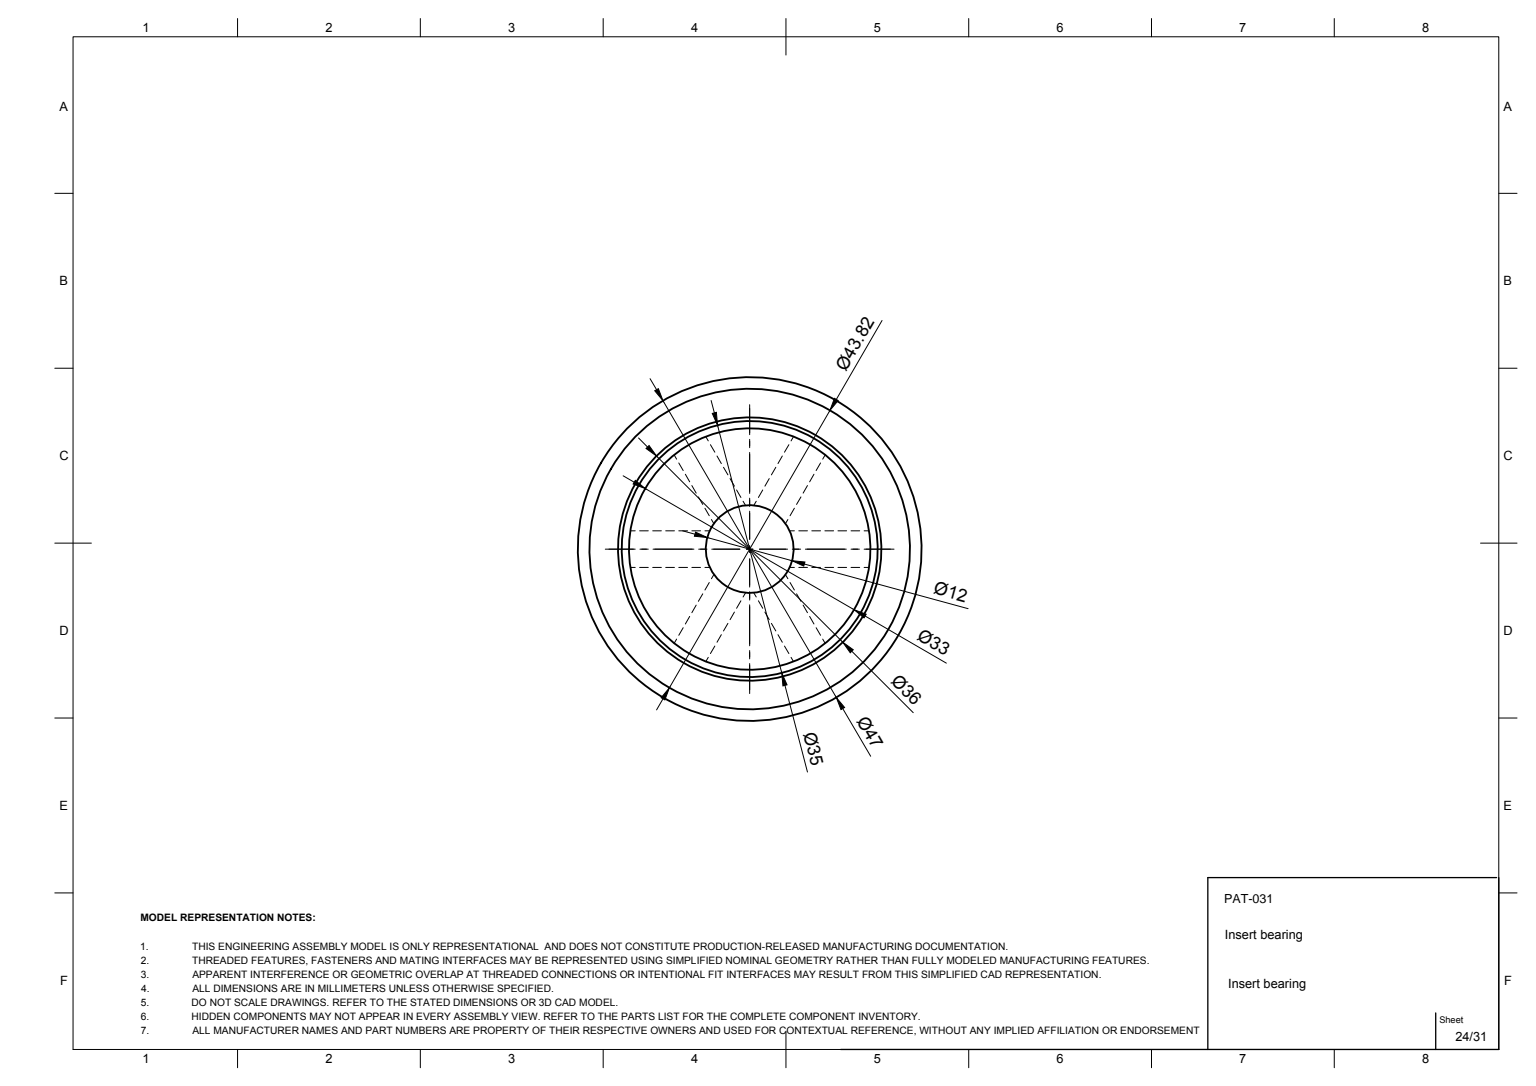
ISO-10303-21;
HEADER;
/* Generated by software containing ST-Developer
 * from STEP Tools, Inc. (www.steptools.com) 
 */

FILE_DESCRIPTION(
/* description */ ('Double-row support with tensioned shaft'),
/* implementation_level */ '2;1');

FILE_NAME(
/* name */ 'Insert bearing.step',
/* time_stamp */ '2026-10-27T10:50:35-07:00',
/* author */ (''),
/* organization */ (''),
/* preprocessor_version */ 'ST-DEVELOPER v20.2',
/* originating_system */ 'Autodesk Translation Framework v15.17.0.0',
/* authorisation */ '');

FILE_SCHEMA (('AUTOMOTIVE_DESIGN { 1 0 10303 214 3 1 1 }'));
ENDSEC;

DATA;
#10=MECHANICAL_DESIGN_GEOMETRIC_PRESENTATION_REPRESENTATION('',(#499,#500),#11559);
#363=B_SPLINE_CURVE_WITH_KNOTS('',3,(#10336,#10337,#10338,#10339,#10340,
#10341,#10342,#10343,#10344,#10345),.UNSPECIFIED.,.F.,.F.,(4,2,2,2,4),(1.13193471301885,
1.22626174930539,1.32058878559194,1.41491753480854,1.50924628402513),
 .UNSPECIFIED.);
#364=B_SPLINE_CURVE_WITH_KNOTS('',3,(#10347,#10348,#10349,#10350,#10351,
#10352,#10353,#10354,#10355,#10356,#10357,#10358,#10359,#10360,#10361,#10362,
#10363,#10364),.UNSPECIFIED.,.F.,.F.,(4,2,2,2,2,2,2,2,4),(0.377311571006283,
0.471638607292829,0.565965643579376,0.66029439279597,0.754623142012565,
0.84895189122916,0.943280640445754,1.0376076767323,1.13193471301885),
 .UNSPECIFIED.);
#365=B_SPLINE_CURVE_WITH_KNOTS('',3,(#10365,#10366,#10367,#10368,#10369,
#10370,#10371,#10372,#10373,#10374),.UNSPECIFIED.,.F.,.F.,(4,2,2,2,4),(1.50924628402513,
1.60357503324173,1.69790378245832,1.79223081874487,1.88655785503141),
 .UNSPECIFIED.);
#366=B_SPLINE_CURVE_WITH_KNOTS('',3,(#10377,#10378,#10379,#10380,#10381,
#10382,#10383,#10384,#10385,#10386,#10387,#10388,#10389,#10390,#10391,#10392,
#10393,#10394,#10395,#10396,#10397,#10398,#10399,#10400,#10401,#10402,#10403,
#10404,#10405,#10406,#10407,#10408,#10409,#10410),.UNSPECIFIED.,.T.,.F.,
(4,2,2,2,2,2,2,2,2,2,2,2,2,2,2,2,4),(0.,0.0955080856649705,0.191016171329941,
0.286408845249646,0.38180151916935,0.477194193089055,0.572586867008759,
0.66809495267373,0.763603038338701,0.859111124003671,0.954619209668642,
1.05001188358835,1.14540455750805,1.24079723142776,1.33618990534746,1.43169799101243,
1.5272060766774),.UNSPECIFIED.);
#367=B_SPLINE_CURVE_WITH_KNOTS('',3,(#10413,#10414,#10415,#10416,#10417,
#10418,#10419,#10420,#10421,#10422,#10423,#10424,#10425,#10426,#10427,#10428,
#10429,#10430,#10431,#10432,#10433,#10434,#10435,#10436,#10437,#10438,#10439,
#10440,#10441,#10442,#10443,#10444,#10445,#10446),.UNSPECIFIED.,.T.,.F.,
(4,2,2,2,2,2,2,2,2,2,2,2,2,2,2,2,4),(0.,0.0955080856649706,0.191016171329941,
0.286408845249646,0.381801519169351,0.477194193089055,0.57258686700876,
0.668094952673731,0.763603038338701,0.859111124003672,0.954619209668642,
1.05001188358835,1.14540455750805,1.24079723142776,1.33618990534746,1.43169799101243,
1.5272060766774),.UNSPECIFIED.);
#368=B_SPLINE_CURVE_WITH_KNOTS('',3,(#10450,#10451,#10452,#10453,#10454,
#10455,#10456,#10457,#10458,#10459),.UNSPECIFIED.,.F.,.F.,(4,2,2,2,4),(1.13193471301885,
1.22626174930539,1.32058878559194,1.41491753480854,1.50924628402513),
 .UNSPECIFIED.);
#369=B_SPLINE_CURVE_WITH_KNOTS('',3,(#10461,#10462,#10463,#10464,#10465,
#10466,#10467,#10468,#10469,#10470,#10471,#10472,#10473,#10474,#10475,#10476,
#10477,#10478),.UNSPECIFIED.,.F.,.F.,(4,2,2,2,2,2,2,2,4),(0.377311571006283,
0.47163860729283,0.565965643579376,0.660294392795971,0.754623142012565,
0.84895189122916,0.943280640445755,1.0376076767323,1.13193471301885),
 .UNSPECIFIED.);
#370=B_SPLINE_CURVE_WITH_KNOTS('',3,(#10479,#10480,#10481,#10482,#10483,
#10484,#10485,#10486,#10487,#10488),.UNSPECIFIED.,.F.,.F.,(4,2,2,2,4),(1.50924628402513,
1.60357503324173,1.69790378245832,1.79223081874487,1.88655785503141),
 .UNSPECIFIED.);
#371=B_SPLINE_CURVE_WITH_KNOTS('',3,(#10497,#10498,#10499,#10500,#10501,
#10502,#10503,#10504,#10505,#10506,#10507,#10508,#10509,#10510,#10511,#10512,
#10513,#10514),.UNSPECIFIED.,.F.,.F.,(4,2,2,2,2,2,2,2,4),(0.377311571006282,
0.471638607292829,0.565965643579376,0.660294392795971,0.754623142012565,
0.84895189122916,0.943280640445754,1.0376076767323,1.13193471301885),
 .UNSPECIFIED.);
#372=B_SPLINE_CURVE_WITH_KNOTS('',3,(#10516,#10517,#10518,#10519,#10520,
#10521,#10522,#10523,#10524,#10525),.UNSPECIFIED.,.F.,.F.,(4,2,2,2,4),(1.13193471301885,
1.22626174930539,1.32058878559194,1.41491753480854,1.50924628402513),
 .UNSPECIFIED.);
#373=B_SPLINE_CURVE_WITH_KNOTS('',3,(#10526,#10527,#10528,#10529,#10530,
#10531,#10532,#10533,#10534,#10535),.UNSPECIFIED.,.F.,.F.,(4,2,2,2,4),(1.50924628402513,
1.60357503324172,1.69790378245832,1.79223081874487,1.88655785503141),
 .UNSPECIFIED.);
#374=B_SPLINE_CURVE_WITH_KNOTS('',3,(#10538,#10539,#10540,#10541,#10542,
#10543,#10544,#10545,#10546,#10547,#10548,#10549,#10550,#10551,#10552,#10553,
#10554,#10555),.UNSPECIFIED.,.F.,.F.,(4,2,2,2,2,2,2,2,4),(0.377311571006283,
0.47163860729283,0.565965643579376,0.660294392795971,0.754623142012565,
0.84895189122916,0.943280640445754,1.0376076767323,1.13193471301885),
 .UNSPECIFIED.);
#375=B_SPLINE_CURVE_WITH_KNOTS('',3,(#10557,#10558,#10559,#10560,#10561,
#10562,#10563,#10564,#10565,#10566),.UNSPECIFIED.,.F.,.F.,(4,2,2,2,4),(1.13193471301885,
1.22626174930539,1.32058878559194,1.41491753480854,1.50924628402513),
 .UNSPECIFIED.);
#376=B_SPLINE_CURVE_WITH_KNOTS('',3,(#10567,#10568,#10569,#10570,#10571,
#10572,#10573,#10574,#10575,#10576),.UNSPECIFIED.,.F.,.F.,(4,2,2,2,4),(1.50924628402513,
1.60357503324173,1.69790378245832,1.79223081874487,1.88655785503141),
 .UNSPECIFIED.);
#377=B_SPLINE_CURVE_WITH_KNOTS('',3,(#10579,#10580,#10581,#10582,#10583,
#10584,#10585,#10586,#10587,#10588,#10589,#10590,#10591,#10592,#10593,#10594,
#10595,#10596),.UNSPECIFIED.,.F.,.F.,(4,2,2,2,2,2,2,2,4),(0.377311571006282,
0.471638607292829,0.565965643579376,0.66029439279597,0.754623142012565,
0.84895189122916,0.943280640445754,1.0376076767323,1.13193471301885),
 .UNSPECIFIED.);
#378=B_SPLINE_CURVE_WITH_KNOTS('',3,(#10598,#10599,#10600,#10601,#10602,
#10603,#10604,#10605,#10606,#10607),.UNSPECIFIED.,.F.,.F.,(4,2,2,2,4),(1.13193471301885,
1.22626174930539,1.32058878559194,1.41491753480854,1.50924628402513),
 .UNSPECIFIED.);
#379=B_SPLINE_CURVE_WITH_KNOTS('',3,(#10608,#10609,#10610,#10611,#10612,
#10613,#10614,#10615,#10616,#10617),.UNSPECIFIED.,.F.,.F.,(4,2,2,2,4),(1.50924628402513,
1.60357503324172,1.69790378245832,1.79223081874487,1.88655785503141),
 .UNSPECIFIED.);
#380=B_SPLINE_CURVE_WITH_KNOTS('',3,(#10620,#10621,#10622,#10623,#10624,
#10625,#10626,#10627,#10628,#10629,#10630,#10631,#10632,#10633,#10634,#10635,
#10636,#10637),.UNSPECIFIED.,.F.,.F.,(4,2,2,2,2,2,2,2,4),(0.377311571006283,
0.471638607292829,0.565965643579376,0.660294392795971,0.754623142012565,
0.84895189122916,0.943280640445755,1.0376076767323,1.13193471301885),
 .UNSPECIFIED.);
#381=B_SPLINE_CURVE_WITH_KNOTS('',3,(#10639,#10640,#10641,#10642,#10643,
#10644,#10645,#10646,#10647,#10648),.UNSPECIFIED.,.F.,.F.,(4,2,2,2,4),(1.13193471301885,
1.22626174930539,1.32058878559194,1.41491753480854,1.50924628402513),
 .UNSPECIFIED.);
#382=B_SPLINE_CURVE_WITH_KNOTS('',3,(#10649,#10650,#10651,#10652,#10653,
#10654,#10655,#10656,#10657,#10658),.UNSPECIFIED.,.F.,.F.,(4,2,2,2,4),(1.50924628402513,
1.60357503324172,1.69790378245832,1.79223081874487,1.88655785503141),
 .UNSPECIFIED.);
#383=B_SPLINE_CURVE_WITH_KNOTS('',3,(#10662,#10663,#10664,#10665,#10666,
#10667,#10668,#10669,#10670,#10671,#10672,#10673,#10674,#10675,#10676,#10677,
#10678,#10679,#10680,#10681,#10682,#10683,#10684,#10685,#10686,#10687,#10688,
#10689,#10690,#10691,#10692,#10693,#10694,#10695),.UNSPECIFIED.,.T.,.F.,
(4,2,2,2,2,2,2,2,2,2,2,2,2,2,2,2,4),(0.,0.0955080856649705,0.191016171329941,
0.286408845249646,0.38180151916935,0.477194193089055,0.572586867008759,
0.66809495267373,0.7636030383387,0.859111124003671,0.954619209668642,1.05001188358835,
1.14540455750805,1.24079723142776,1.33618990534746,1.43169799101243,1.5272060766774),
 .UNSPECIFIED.);
#384=B_SPLINE_CURVE_WITH_KNOTS('',3,(#10698,#10699,#10700,#10701,#10702,
#10703,#10704,#10705,#10706,#10707,#10708,#10709,#10710,#10711,#10712,#10713,
#10714,#10715,#10716,#10717,#10718,#10719,#10720,#10721,#10722,#10723,#10724,
#10725,#10726,#10727,#10728,#10729,#10730,#10731),.UNSPECIFIED.,.T.,.F.,
(4,2,2,2,2,2,2,2,2,2,2,2,2,2,2,2,4),(0.,0.0955080856649706,0.191016171329941,
0.286408845249646,0.381801519169351,0.477194193089055,0.57258686700876,
0.668094952673731,0.763603038338701,0.859111124003672,0.954619209668642,
1.05001188358835,1.14540455750805,1.24079723142776,1.33618990534746,1.43169799101243,
1.5272060766774),.UNSPECIFIED.);
#385=B_SPLINE_CURVE_WITH_KNOTS('',3,(#10736,#10737,#10738,#10739,#10740,
#10741,#10742,#10743,#10744,#10745,#10746,#10747,#10748,#10749,#10750,#10751,
#10752,#10753,#10754,#10755,#10756,#10757,#10758,#10759,#10760,#10761,#10762,
#10763,#10764,#10765,#10766,#10767,#10768,#10769),.UNSPECIFIED.,.T.,.F.,
(4,2,2,2,2,2,2,2,2,2,2,2,2,2,2,2,4),(0.,0.0955080856649705,0.191016171329941,
0.286408845249646,0.38180151916935,0.477194193089055,0.572586867008759,
0.66809495267373,0.7636030383387,0.859111124003671,0.954619209668642,1.05001188358835,
1.14540455750805,1.24079723142776,1.33618990534746,1.43169799101243,1.5272060766774),
 .UNSPECIFIED.);
#386=B_SPLINE_CURVE_WITH_KNOTS('',3,(#10772,#10773,#10774,#10775,#10776,
#10777,#10778,#10779,#10780,#10781,#10782,#10783,#10784,#10785,#10786,#10787,
#10788,#10789,#10790,#10791,#10792,#10793,#10794,#10795,#10796,#10797,#10798,
#10799,#10800,#10801,#10802,#10803,#10804,#10805),.UNSPECIFIED.,.T.,.F.,
(4,2,2,2,2,2,2,2,2,2,2,2,2,2,2,2,4),(0.,0.0955080856649706,0.191016171329941,
0.286408845249646,0.381801519169351,0.477194193089055,0.57258686700876,
0.668094952673731,0.763603038338701,0.859111124003672,0.954619209668642,
1.05001188358835,1.14540455750805,1.24079723142776,1.33618990534746,1.43169799101243,
1.5272060766774),.UNSPECIFIED.);
#392=SPHERICAL_SURFACE('',#7083,2.35);
#435=SHAPE_REPRESENTATION_RELATIONSHIP('SRR','None',#11744,#467);
#467=ADVANCED_BREP_SHAPE_REPRESENTATION('',(#530,#531),#11546);
#499=STYLED_ITEM('',(#11967),#530);
#500=STYLED_ITEM('',(#11967),#531);
#530=MANIFOLD_SOLID_BREP('Body1',#6346);
#531=MANIFOLD_SOLID_BREP('Body2',#6347);
#629=FACE_BOUND('',#1568,.T.);
#630=FACE_BOUND('',#1570,.T.);
#631=FACE_BOUND('',#1571,.T.);
#632=FACE_BOUND('',#1573,.T.);
#633=FACE_BOUND('',#1577,.T.);
#634=FACE_BOUND('',#1578,.T.);
#635=FACE_BOUND('',#1579,.T.);
#636=FACE_BOUND('',#1580,.T.);
#637=FACE_BOUND('',#1581,.T.);
#638=FACE_BOUND('',#1582,.T.);
#639=FACE_BOUND('',#1588,.T.);
#640=FACE_BOUND('',#1590,.T.);
#641=FACE_BOUND('',#1593,.T.);
#642=FACE_BOUND('',#1595,.T.);
#643=FACE_BOUND('',#1596,.T.);
#644=FACE_BOUND('',#1597,.T.);
#645=FACE_BOUND('',#1598,.T.);
#646=FACE_BOUND('',#1599,.T.);
#647=FACE_BOUND('',#1600,.T.);
#834=PLANE('',#7081);
#835=PLANE('',#7086);
#836=PLANE('',#7096);
#837=PLANE('',#7098);
#838=PLANE('',#7102);
#1135=FACE_OUTER_BOUND('',#1566,.T.);
#1136=FACE_OUTER_BOUND('',#1567,.T.);
#1137=FACE_OUTER_BOUND('',#1569,.T.);
#1138=FACE_OUTER_BOUND('',#1572,.T.);
#1139=FACE_OUTER_BOUND('',#1574,.T.);
#1140=FACE_OUTER_BOUND('',#1575,.T.);
#1141=FACE_OUTER_BOUND('',#1576,.T.);
#1142=FACE_OUTER_BOUND('',#1583,.T.);
#1143=FACE_OUTER_BOUND('',#1584,.T.);
#1144=FACE_OUTER_BOUND('',#1585,.T.);
#1145=FACE_OUTER_BOUND('',#1586,.T.);
#1146=FACE_OUTER_BOUND('',#1587,.T.);
#1147=FACE_OUTER_BOUND('',#1589,.T.);
#1148=FACE_OUTER_BOUND('',#1591,.T.);
#1149=FACE_OUTER_BOUND('',#1592,.T.);
#1150=FACE_OUTER_BOUND('',#1594,.T.);
#1566=EDGE_LOOP('',(#5340,#5341,#5342,#5343));
#1567=EDGE_LOOP('',(#5344));
#1568=EDGE_LOOP('',(#5345));
#1569=EDGE_LOOP('',(#5346,#5347));
#1570=EDGE_LOOP('',(#5348));
#1571=EDGE_LOOP('',(#5349));
#1572=EDGE_LOOP('',(#5350));
#1573=EDGE_LOOP('',(#5351));
#1574=EDGE_LOOP('',(#5352,#5353,#5354,#5355,#5356,#5357));
#1575=EDGE_LOOP('',(#5358,#5359,#5360,#5361,#5362,#5363));
#1576=EDGE_LOOP('',(#5364,#5365,#5366,#5367));
#1577=EDGE_LOOP('',(#5368,#5369,#5370));
#1578=EDGE_LOOP('',(#5371,#5372,#5373));
#1579=EDGE_LOOP('',(#5374,#5375,#5376));
#1580=EDGE_LOOP('',(#5377,#5378,#5379));
#1581=EDGE_LOOP('',(#5380,#5381,#5382));
#1582=EDGE_LOOP('',(#5383,#5384,#5385));
#1583=EDGE_LOOP('',(#5386,#5387,#5388,#5389,#5390,#5391));
#1584=EDGE_LOOP('',(#5392,#5393,#5394,#5395,#5396,#5397));
#1585=EDGE_LOOP('',(#5398,#5399,#5400,#5401,#5402,#5403));
#1586=EDGE_LOOP('',(#5404,#5405,#5406,#5407,#5408,#5409));
#1587=EDGE_LOOP('',(#5410));
#1588=EDGE_LOOP('',(#5411));
#1589=EDGE_LOOP('',(#5412));
#1590=EDGE_LOOP('',(#5413));
#1591=EDGE_LOOP('',(#5414,#5415,#5416,#5417));
#1592=EDGE_LOOP('',(#5418));
#1593=EDGE_LOOP('',(#5419));
#1594=EDGE_LOOP('',(#5420,#5421,#5422,#5423));
#1595=EDGE_LOOP('',(#5424));
#1596=EDGE_LOOP('',(#5425));
#1597=EDGE_LOOP('',(#5426));
#1598=EDGE_LOOP('',(#5427));
#1599=EDGE_LOOP('',(#5428));
#1600=EDGE_LOOP('',(#5429));
#2124=LINE('',#10321,#2671);
#2125=LINE('',#10376,#2672);
#2126=LINE('',#10448,#2673);
#2127=LINE('',#10493,#2674);
#2128=LINE('',#10661,#2675);
#2129=LINE('',#10732,#2676);
#2130=LINE('',#10735,#2677);
#2131=LINE('',#10806,#2678);
#2132=LINE('',#10816,#2679);
#2133=LINE('',#10821,#2680);
#2671=VECTOR('',#8487,1.8);
#2672=VECTOR('',#8504,0.25);
#2673=VECTOR('',#8507,0.25);
#2674=VECTOR('',#8512,1.65);
#2675=VECTOR('',#8517,0.25);
#2676=VECTOR('',#8520,0.25);
#2677=VECTOR('',#8523,0.25);
#2678=VECTOR('',#8526,0.25);
#2679=VECTOR('',#8539,1.75);
#2680=VECTOR('',#8546,0.6);
#2957=CIRCLE('',#7079,1.8);
#2958=CIRCLE('',#7080,1.8);
#2959=CIRCLE('',#7082,2.19089023002066);
#2960=CIRCLE('',#7084,2.35);
#2961=CIRCLE('',#7085,2.19089023002066);
#2962=CIRCLE('',#7090,1.65);
#2963=CIRCLE('',#7091,1.65);
#2964=CIRCLE('',#7097,0.6);
#2965=CIRCLE('',#7099,1.75);
#2966=CIRCLE('',#7101,1.75);
#2967=CIRCLE('',#7103,0.6);
#3363=VERTEX_POINT('',#10318);
#3364=VERTEX_POINT('',#10320);
#3365=VERTEX_POINT('',#10324);
#3366=VERTEX_POINT('',#10327);
#3367=VERTEX_POINT('',#10328);
#3368=VERTEX_POINT('',#10330);
#3369=VERTEX_POINT('',#10334);
#3370=VERTEX_POINT('',#10335);
#3371=VERTEX_POINT('',#10346);
#3372=VERTEX_POINT('',#10375);
#3373=VERTEX_POINT('',#10412);
#3374=VERTEX_POINT('',#10447);
#3375=VERTEX_POINT('',#10449);
#3376=VERTEX_POINT('',#10460);
#3377=VERTEX_POINT('',#10490);
#3378=VERTEX_POINT('',#10492);
#3379=VERTEX_POINT('',#10495);
#3380=VERTEX_POINT('',#10496);
#3381=VERTEX_POINT('',#10515);
#3382=VERTEX_POINT('',#10536);
#3383=VERTEX_POINT('',#10537);
#3384=VERTEX_POINT('',#10556);
#3385=VERTEX_POINT('',#10577);
#3386=VERTEX_POINT('',#10578);
#3387=VERTEX_POINT('',#10597);
#3388=VERTEX_POINT('',#10618);
#3389=VERTEX_POINT('',#10619);
#3390=VERTEX_POINT('',#10638);
#3391=VERTEX_POINT('',#10660);
#3392=VERTEX_POINT('',#10697);
#3393=VERTEX_POINT('',#10734);
#3394=VERTEX_POINT('',#10771);
#3395=VERTEX_POINT('',#10808);
#3396=VERTEX_POINT('',#10811);
#3397=VERTEX_POINT('',#10814);
#3398=VERTEX_POINT('',#10818);
#4055=EDGE_CURVE('',#3363,#3363,#2957,.T.);
#4056=EDGE_CURVE('',#3363,#3364,#2124,.T.);
#4057=EDGE_CURVE('',#3364,#3364,#2958,.T.);
#4058=EDGE_CURVE('',#3365,#3365,#2959,.T.);
#4059=EDGE_CURVE('',#3366,#3367,#2960,.T.);
#4060=EDGE_CURVE('',#3368,#3368,#2961,.T.);
#4061=EDGE_CURVE('',#3369,#3370,#363,.T.);
#4062=EDGE_CURVE('',#3371,#3369,#364,.T.);
#4063=EDGE_CURVE('',#3370,#3371,#365,.T.);
#4064=EDGE_CURVE('',#3370,#3372,#2125,.T.);
#4065=EDGE_CURVE('',#3372,#3372,#366,.T.);
#4066=EDGE_CURVE('',#3373,#3373,#367,.T.);
#4067=EDGE_CURVE('',#3373,#3374,#2126,.T.);
#4068=EDGE_CURVE('',#3375,#3374,#368,.T.);
#4069=EDGE_CURVE('',#3376,#3375,#369,.T.);
#4070=EDGE_CURVE('',#3374,#3376,#370,.T.);
#4071=EDGE_CURVE('',#3377,#3377,#2962,.T.);
#4072=EDGE_CURVE('',#3377,#3378,#2127,.T.);
#4073=EDGE_CURVE('',#3378,#3378,#2963,.T.);
#4074=EDGE_CURVE('',#3379,#3380,#371,.T.);
#4075=EDGE_CURVE('',#3380,#3381,#372,.T.);
#4076=EDGE_CURVE('',#3381,#3379,#373,.T.);
#4077=EDGE_CURVE('',#3382,#3383,#374,.T.);
#4078=EDGE_CURVE('',#3383,#3384,#375,.T.);
#4079=EDGE_CURVE('',#3384,#3382,#376,.T.);
#4080=EDGE_CURVE('',#3385,#3386,#377,.T.);
#4081=EDGE_CURVE('',#3386,#3387,#378,.T.);
#4082=EDGE_CURVE('',#3387,#3385,#379,.T.);
#4083=EDGE_CURVE('',#3388,#3389,#380,.T.);
#4084=EDGE_CURVE('',#3389,#3390,#381,.T.);
#4085=EDGE_CURVE('',#3390,#3388,#382,.T.);
#4086=EDGE_CURVE('',#3381,#3391,#2128,.T.);
#4087=EDGE_CURVE('',#3391,#3391,#383,.T.);
#4088=EDGE_CURVE('',#3392,#3392,#384,.T.);
#4089=EDGE_CURVE('',#3392,#3384,#2129,.T.);
#4090=EDGE_CURVE('',#3387,#3393,#2130,.T.);
#4091=EDGE_CURVE('',#3393,#3393,#385,.T.);
#4092=EDGE_CURVE('',#3394,#3394,#386,.T.);
#4093=EDGE_CURVE('',#3394,#3390,#2131,.T.);
#4094=EDGE_CURVE('',#3395,#3395,#2964,.T.);
#4095=EDGE_CURVE('',#3396,#3396,#2965,.T.);
#4096=EDGE_CURVE('',#3397,#3397,#2966,.T.);
#4097=EDGE_CURVE('',#3397,#3396,#2132,.T.);
#4098=EDGE_CURVE('',#3398,#3398,#2967,.T.);
#4099=EDGE_CURVE('',#3398,#3395,#2133,.T.);
#5340=ORIENTED_EDGE('',*,*,#4055,.T.);
#5341=ORIENTED_EDGE('',*,*,#4056,.T.);
#5342=ORIENTED_EDGE('',*,*,#4057,.F.);
#5343=ORIENTED_EDGE('',*,*,#4056,.F.);
#5344=ORIENTED_EDGE('',*,*,#4058,.F.);
#5345=ORIENTED_EDGE('',*,*,#4057,.T.);
#5346=ORIENTED_EDGE('',*,*,#4059,.T.);
#5347=ORIENTED_EDGE('',*,*,#4059,.F.);
#5348=ORIENTED_EDGE('',*,*,#4058,.T.);
#5349=ORIENTED_EDGE('',*,*,#4060,.F.);
#5350=ORIENTED_EDGE('',*,*,#4060,.T.);
#5351=ORIENTED_EDGE('',*,*,#4055,.F.);
#5352=ORIENTED_EDGE('',*,*,#4061,.F.);
#5353=ORIENTED_EDGE('',*,*,#4062,.F.);
#5354=ORIENTED_EDGE('',*,*,#4063,.F.);
#5355=ORIENTED_EDGE('',*,*,#4064,.T.);
#5356=ORIENTED_EDGE('',*,*,#4065,.F.);
#5357=ORIENTED_EDGE('',*,*,#4064,.F.);
#5358=ORIENTED_EDGE('',*,*,#4066,.F.);
#5359=ORIENTED_EDGE('',*,*,#4067,.T.);
#5360=ORIENTED_EDGE('',*,*,#4068,.F.);
#5361=ORIENTED_EDGE('',*,*,#4069,.F.);
#5362=ORIENTED_EDGE('',*,*,#4070,.F.);
#5363=ORIENTED_EDGE('',*,*,#4067,.F.);
#5364=ORIENTED_EDGE('',*,*,#4071,.F.);
#5365=ORIENTED_EDGE('',*,*,#4072,.T.);
#5366=ORIENTED_EDGE('',*,*,#4073,.T.);
#5367=ORIENTED_EDGE('',*,*,#4072,.F.);
#5368=ORIENTED_EDGE('',*,*,#4062,.T.);
#5369=ORIENTED_EDGE('',*,*,#4061,.T.);
#5370=ORIENTED_EDGE('',*,*,#4063,.T.);
#5371=ORIENTED_EDGE('',*,*,#4069,.T.);
#5372=ORIENTED_EDGE('',*,*,#4068,.T.);
#5373=ORIENTED_EDGE('',*,*,#4070,.T.);
#5374=ORIENTED_EDGE('',*,*,#4074,.T.);
#5375=ORIENTED_EDGE('',*,*,#4075,.T.);
#5376=ORIENTED_EDGE('',*,*,#4076,.T.);
#5377=ORIENTED_EDGE('',*,*,#4077,.T.);
#5378=ORIENTED_EDGE('',*,*,#4078,.T.);
#5379=ORIENTED_EDGE('',*,*,#4079,.T.);
#5380=ORIENTED_EDGE('',*,*,#4080,.T.);
#5381=ORIENTED_EDGE('',*,*,#4081,.T.);
#5382=ORIENTED_EDGE('',*,*,#4082,.T.);
#5383=ORIENTED_EDGE('',*,*,#4083,.T.);
#5384=ORIENTED_EDGE('',*,*,#4084,.T.);
#5385=ORIENTED_EDGE('',*,*,#4085,.T.);
#5386=ORIENTED_EDGE('',*,*,#4075,.F.);
#5387=ORIENTED_EDGE('',*,*,#4074,.F.);
#5388=ORIENTED_EDGE('',*,*,#4076,.F.);
#5389=ORIENTED_EDGE('',*,*,#4086,.T.);
#5390=ORIENTED_EDGE('',*,*,#4087,.F.);
#5391=ORIENTED_EDGE('',*,*,#4086,.F.);
#5392=ORIENTED_EDGE('',*,*,#4088,.F.);
#5393=ORIENTED_EDGE('',*,*,#4089,.T.);
#5394=ORIENTED_EDGE('',*,*,#4078,.F.);
#5395=ORIENTED_EDGE('',*,*,#4077,.F.);
#5396=ORIENTED_EDGE('',*,*,#4079,.F.);
#5397=ORIENTED_EDGE('',*,*,#4089,.F.);
#5398=ORIENTED_EDGE('',*,*,#4081,.F.);
#5399=ORIENTED_EDGE('',*,*,#4080,.F.);
#5400=ORIENTED_EDGE('',*,*,#4082,.F.);
#5401=ORIENTED_EDGE('',*,*,#4090,.T.);
#5402=ORIENTED_EDGE('',*,*,#4091,.F.);
#5403=ORIENTED_EDGE('',*,*,#4090,.F.);
#5404=ORIENTED_EDGE('',*,*,#4092,.F.);
#5405=ORIENTED_EDGE('',*,*,#4093,.T.);
#5406=ORIENTED_EDGE('',*,*,#4084,.F.);
#5407=ORIENTED_EDGE('',*,*,#4083,.F.);
#5408=ORIENTED_EDGE('',*,*,#4085,.F.);
#5409=ORIENTED_EDGE('',*,*,#4093,.F.);
#5410=ORIENTED_EDGE('',*,*,#4073,.F.);
#5411=ORIENTED_EDGE('',*,*,#4094,.T.);
#5412=ORIENTED_EDGE('',*,*,#4095,.F.);
#5413=ORIENTED_EDGE('',*,*,#4071,.T.);
#5414=ORIENTED_EDGE('',*,*,#4096,.F.);
#5415=ORIENTED_EDGE('',*,*,#4097,.T.);
#5416=ORIENTED_EDGE('',*,*,#4095,.T.);
#5417=ORIENTED_EDGE('',*,*,#4097,.F.);
#5418=ORIENTED_EDGE('',*,*,#4096,.T.);
#5419=ORIENTED_EDGE('',*,*,#4098,.F.);
#5420=ORIENTED_EDGE('',*,*,#4098,.T.);
#5421=ORIENTED_EDGE('',*,*,#4099,.T.);
#5422=ORIENTED_EDGE('',*,*,#4094,.F.);
#5423=ORIENTED_EDGE('',*,*,#4099,.F.);
#5424=ORIENTED_EDGE('',*,*,#4066,.T.);
#5425=ORIENTED_EDGE('',*,*,#4065,.T.);
#5426=ORIENTED_EDGE('',*,*,#4088,.T.);
#5427=ORIENTED_EDGE('',*,*,#4087,.T.);
#5428=ORIENTED_EDGE('',*,*,#4092,.T.);
#5429=ORIENTED_EDGE('',*,*,#4091,.T.);
#5946=CYLINDRICAL_SURFACE('',#7078,1.8);
#5947=CYLINDRICAL_SURFACE('',#7087,0.25);
#5948=CYLINDRICAL_SURFACE('',#7088,0.25);
#5949=CYLINDRICAL_SURFACE('',#7089,1.65);
#5950=CYLINDRICAL_SURFACE('',#7092,0.25);
#5951=CYLINDRICAL_SURFACE('',#7093,0.25);
#5952=CYLINDRICAL_SURFACE('',#7094,0.25);
#5953=CYLINDRICAL_SURFACE('',#7095,0.25);
#5954=CYLINDRICAL_SURFACE('',#7100,1.75);
#5955=CYLINDRICAL_SURFACE('',#7104,0.6);
#6198=ADVANCED_FACE('',(#1135),#5946,.F.);
#6199=ADVANCED_FACE('',(#1136,#629),#834,.T.);
#6200=ADVANCED_FACE('',(#1137,#630,#631),#392,.T.);
#6201=ADVANCED_FACE('',(#1138,#632),#835,.T.);
#6202=ADVANCED_FACE('',(#1139),#5947,.F.);
#6203=ADVANCED_FACE('',(#1140),#5948,.F.);
#6204=ADVANCED_FACE('',(#1141,#633,#634,#635,#636,#637,#638),#5949,.T.);
#6205=ADVANCED_FACE('',(#1142),#5950,.F.);
#6206=ADVANCED_FACE('',(#1143),#5951,.F.);
#6207=ADVANCED_FACE('',(#1144),#5952,.F.);
#6208=ADVANCED_FACE('',(#1145),#5953,.F.);
#6209=ADVANCED_FACE('',(#1146,#639),#836,.T.);
#6210=ADVANCED_FACE('',(#1147,#640),#837,.T.);
#6211=ADVANCED_FACE('',(#1148),#5954,.T.);
#6212=ADVANCED_FACE('',(#1149,#641),#838,.T.);
#6213=ADVANCED_FACE('',(#1150,#642,#643,#644,#645,#646,#647),#5955,.F.);
#6346=CLOSED_SHELL('',(#6198,#6199,#6200,#6201));
#6347=CLOSED_SHELL('',(#6202,#6203,#6204,#6205,#6206,#6207,#6208,#6209,
#6210,#6211,#6212,#6213));
#7077=AXIS2_PLACEMENT_3D('',#10316,#8481,#8482);
#7078=AXIS2_PLACEMENT_3D('',#10317,#8483,#8484);
#7079=AXIS2_PLACEMENT_3D('',#10319,#8485,#8486);
#7080=AXIS2_PLACEMENT_3D('',#10322,#8488,#8489);
#7081=AXIS2_PLACEMENT_3D('',#10323,#8490,#8491);
#7082=AXIS2_PLACEMENT_3D('',#10325,#8492,#8493);
#7083=AXIS2_PLACEMENT_3D('',#10326,#8494,#8495);
#7084=AXIS2_PLACEMENT_3D('',#10329,#8496,#8497);
#7085=AXIS2_PLACEMENT_3D('',#10331,#8498,#8499);
#7086=AXIS2_PLACEMENT_3D('',#10332,#8500,#8501);
#7087=AXIS2_PLACEMENT_3D('',#10333,#8502,#8503);
#7088=AXIS2_PLACEMENT_3D('',#10411,#8505,#8506);
#7089=AXIS2_PLACEMENT_3D('',#10489,#8508,#8509);
#7090=AXIS2_PLACEMENT_3D('',#10491,#8510,#8511);
#7091=AXIS2_PLACEMENT_3D('',#10494,#8513,#8514);
#7092=AXIS2_PLACEMENT_3D('',#10659,#8515,#8516);
#7093=AXIS2_PLACEMENT_3D('',#10696,#8518,#8519);
#7094=AXIS2_PLACEMENT_3D('',#10733,#8521,#8522);
#7095=AXIS2_PLACEMENT_3D('',#10770,#8524,#8525);
#7096=AXIS2_PLACEMENT_3D('',#10807,#8527,#8528);
#7097=AXIS2_PLACEMENT_3D('',#10809,#8529,#8530);
#7098=AXIS2_PLACEMENT_3D('',#10810,#8531,#8532);
#7099=AXIS2_PLACEMENT_3D('',#10812,#8533,#8534);
#7100=AXIS2_PLACEMENT_3D('',#10813,#8535,#8536);
#7101=AXIS2_PLACEMENT_3D('',#10815,#8537,#8538);
#7102=AXIS2_PLACEMENT_3D('',#10817,#8540,#8541);
#7103=AXIS2_PLACEMENT_3D('',#10819,#8542,#8543);
#7104=AXIS2_PLACEMENT_3D('',#10820,#8544,#8545);
#8481=DIRECTION('axis',(0.,0.,1.));
#8482=DIRECTION('refdir',(1.,0.,0.));
#8483=DIRECTION('center_axis',(0.,-1.,0.));
#8484=DIRECTION('ref_axis',(1.,0.,0.));
#8485=DIRECTION('center_axis',(0.,-1.,0.));
#8486=DIRECTION('ref_axis',(1.,0.,0.));
#8487=DIRECTION('',(0.,1.,0.));
#8488=DIRECTION('center_axis',(0.,-1.,0.));
#8489=DIRECTION('ref_axis',(1.,0.,0.));
#8490=DIRECTION('center_axis',(0.,1.,0.));
#8491=DIRECTION('ref_axis',(0.,0.,1.));
#8492=DIRECTION('center_axis',(0.,-1.,0.));
#8493=DIRECTION('ref_axis',(1.,0.,0.));
#8494=DIRECTION('center_axis',(6.12323399573677E-17,0.,1.));
#8495=DIRECTION('ref_axis',(1.,0.,0.));
#8496=DIRECTION('center_axis',(1.22464679914735E-16,-1.,0.));
#8497=DIRECTION('ref_axis',(-1.,-1.22464679914735E-16,0.));
#8498=DIRECTION('center_axis',(0.,-1.,0.));
#8499=DIRECTION('ref_axis',(1.,0.,0.));
#8500=DIRECTION('center_axis',(0.,-1.,0.));
#8501=DIRECTION('ref_axis',(0.,0.,-1.));
#8502=DIRECTION('center_axis',(-0.866025403784438,0.,-0.5));
#8503=DIRECTION('ref_axis',(-0.5,0.,0.866025403784438));
#8504=DIRECTION('',(-0.866025403784438,0.,-0.5));
#8505=DIRECTION('center_axis',(-0.866025403784438,0.,-0.5));
#8506=DIRECTION('ref_axis',(-0.5,0.,0.866025403784438));
#8507=DIRECTION('',(-0.866025403784438,0.,-0.5));
#8508=DIRECTION('center_axis',(0.,-1.,0.));
#8509=DIRECTION('ref_axis',(1.,0.,0.));
#8510=DIRECTION('center_axis',(0.,-1.,0.));
#8511=DIRECTION('ref_axis',(1.,0.,0.));
#8512=DIRECTION('',(0.,1.,0.));
#8513=DIRECTION('center_axis',(0.,-1.,0.));
#8514=DIRECTION('ref_axis',(1.,0.,0.));
#8515=DIRECTION('center_axis',(0.866025403784439,0.,-0.5));
#8516=DIRECTION('ref_axis',(-0.5,0.,-0.866025403784439));
#8517=DIRECTION('',(0.866025403784439,0.,-0.5));
#8518=DIRECTION('center_axis',(0.866025403784439,0.,-0.5));
#8519=DIRECTION('ref_axis',(-0.5,0.,-0.866025403784439));
#8520=DIRECTION('',(0.866025403784439,0.,-0.5));
#8521=DIRECTION('center_axis',(0.,0.,1.));
#8522=DIRECTION('ref_axis',(1.,0.,0.));
#8523=DIRECTION('',(0.,0.,1.));
#8524=DIRECTION('center_axis',(0.,0.,1.));
#8525=DIRECTION('ref_axis',(1.,0.,0.));
#8526=DIRECTION('',(0.,0.,1.));
#8527=DIRECTION('center_axis',(0.,1.,0.));
#8528=DIRECTION('ref_axis',(0.,0.,1.));
#8529=DIRECTION('center_axis',(0.,-1.,0.));
#8530=DIRECTION('ref_axis',(1.,0.,0.));
#8531=DIRECTION('center_axis',(0.,1.,0.));
#8532=DIRECTION('ref_axis',(0.,0.,1.));
#8533=DIRECTION('center_axis',(0.,-1.,0.));
#8534=DIRECTION('ref_axis',(1.,0.,0.));
#8535=DIRECTION('center_axis',(0.,-1.,0.));
#8536=DIRECTION('ref_axis',(1.,0.,0.));
#8537=DIRECTION('center_axis',(0.,-1.,0.));
#8538=DIRECTION('ref_axis',(1.,0.,0.));
#8539=DIRECTION('',(0.,1.,0.));
#8540=DIRECTION('center_axis',(0.,-1.,0.));
#8541=DIRECTION('ref_axis',(0.,0.,-1.));
#8542=DIRECTION('center_axis',(0.,-1.,0.));
#8543=DIRECTION('ref_axis',(1.,0.,0.));
#8544=DIRECTION('center_axis',(0.,-1.,0.));
#8545=DIRECTION('ref_axis',(1.,0.,0.));
#8546=DIRECTION('',(0.,1.,0.));
#10316=CARTESIAN_POINT('',(0.,0.,0.));
#10317=CARTESIAN_POINT('Origin',(0.,0.,0.));
#10318=CARTESIAN_POINT('',(-1.8,-0.85,-2.20436423846524E-16));
#10319=CARTESIAN_POINT('Origin',(0.,-0.85,0.));
#10320=CARTESIAN_POINT('',(-1.8,0.85,-2.20436423846524E-16));
#10321=CARTESIAN_POINT('',(-1.8,0.,-2.20436423846524E-16));
#10322=CARTESIAN_POINT('Origin',(0.,0.85,0.));
#10323=CARTESIAN_POINT('Origin',(2.19089023002066,0.85,0.));
#10324=CARTESIAN_POINT('',(2.19089023002066,0.85,0.));
#10325=CARTESIAN_POINT('Origin',(0.,0.85,0.));
#10326=CARTESIAN_POINT('Origin',(3.99680288865056E-15,0.,0.));
#10327=CARTESIAN_POINT('',(3.85290688975075E-15,-1.76221774462768E-32,2.35));
#10328=CARTESIAN_POINT('',(3.85290688975075E-15,-1.76221774462768E-32,-2.35));
#10329=CARTESIAN_POINT('Origin',(3.99680288865056E-15,0.,0.));
#10330=CARTESIAN_POINT('',(2.19089023002066,-0.85,0.));
#10331=CARTESIAN_POINT('Origin',(0.,-0.85,0.));
#10332=CARTESIAN_POINT('Origin',(1.8,-0.85,0.));
#10333=CARTESIAN_POINT('Origin',(0.,1.55,0.));
#10334=CARTESIAN_POINT('',(1.42894191624432,1.8,0.825000000000001));
#10335=CARTESIAN_POINT('',(1.53744468918255,1.55,0.598968970568896));
#10336=CARTESIAN_POINT('Ctrl Pts',(1.42894191624432,1.8,0.825000000000001));
#10337=CARTESIAN_POINT('Ctrl Pts',(1.44466308895875,1.8,0.797770130104052));
#10338=CARTESIAN_POINT('Ctrl Pts',(1.46055812562105,1.79370633789704,0.768258557763732));
#10339=CARTESIAN_POINT('Ctrl Pts',(1.48824888379079,1.76817777258318,0.713138492740816));
#10340=CARTESIAN_POINT('Ctrl Pts',(1.50008999307766,1.74894552961493,0.687551581002689));
#10341=CARTESIAN_POINT('Ctrl Pts',(1.51812136280714,1.70460745840382,0.646764802471699));
#10342=CARTESIAN_POINT('Ctrl Pts',(1.52552758004446,1.67652816181843,0.628833667319578));
#10343=CARTESIAN_POINT('Ctrl Pts',(1.53516661651472,1.61494799959182,0.604921184808251));
#10344=CARTESIAN_POINT('Ctrl Pts',(1.53744468918255,1.58144291640553,0.598968970568896));
#10345=CARTESIAN_POINT('Ctrl Pts',(1.53744468918255,1.55,0.598968970568896));
#10346=CARTESIAN_POINT('',(1.42894191624432,1.3,0.825000000000001));
#10347=CARTESIAN_POINT('Ctrl Pts',(1.42894191624432,1.3,0.825000000000001));
#10348=CARTESIAN_POINT('Ctrl Pts',(1.4132207435299,1.3,0.852229869895949));
#10349=CARTESIAN_POINT('Ctrl Pts',(1.39561049050871,1.30629366210296,0.880751161609749));
#10350=CARTESIAN_POINT('Ctrl Pts',(1.36172049302549,1.33182222741682,0.932292094146256));
#10351=CARTESIAN_POINT('Ctrl Pts',(1.34548213209931,1.35105447038507,0.955340251466734));
#10352=CARTESIAN_POINT('Ctrl Pts',(1.31917543061769,1.39539254159618,0.99134926498299));
#10353=CARTESIAN_POINT('Ctrl Pts',(1.30734972067592,1.42347183818157,1.00672880483252));
#10354=CARTESIAN_POINT('Ctrl Pts',(1.29146042158868,1.48505200040818,1.02703269653942));
#10355=CARTESIAN_POINT('Ctrl Pts',(1.28744468918255,1.51855708359447,1.03198167246111));
#10356=CARTESIAN_POINT('Ctrl Pts',(1.28744468918255,1.58144291640553,1.03198167246111));
#10357=CARTESIAN_POINT('Ctrl Pts',(1.29146042158868,1.61494799959182,1.02703269653942));
#10358=CARTESIAN_POINT('Ctrl Pts',(1.30734972067592,1.67652816181843,1.00672880483252));
#10359=CARTESIAN_POINT('Ctrl Pts',(1.31917543061769,1.70460745840382,0.991349264982991));
#10360=CARTESIAN_POINT('Ctrl Pts',(1.34548213209931,1.74894552961493,0.955340251466735));
#10361=CARTESIAN_POINT('Ctrl Pts',(1.36172049302549,1.76817777258318,0.932292094146256));
#10362=CARTESIAN_POINT('Ctrl Pts',(1.39561049050871,1.79370633789704,0.880751161609749));
#10363=CARTESIAN_POINT('Ctrl Pts',(1.4132207435299,1.8,0.85222986989595));
#10364=CARTESIAN_POINT('Ctrl Pts',(1.42894191624432,1.8,0.825000000000001));
#10365=CARTESIAN_POINT('Ctrl Pts',(1.53744468918255,1.55,0.598968970568896));
#10366=CARTESIAN_POINT('Ctrl Pts',(1.53744468918255,1.51855708359447,0.598968970568896));
#10367=CARTESIAN_POINT('Ctrl Pts',(1.53516661651472,1.48505200040818,0.60492118480825));
#10368=CARTESIAN_POINT('Ctrl Pts',(1.52552758004446,1.42347183818157,0.628833667319578));
#10369=CARTESIAN_POINT('Ctrl Pts',(1.51812136280714,1.39539254159618,0.646764802471699));
#10370=CARTESIAN_POINT('Ctrl Pts',(1.50008999307766,1.35105447038507,0.687551581002689));
#10371=CARTESIAN_POINT('Ctrl Pts',(1.48824888379079,1.33182222741682,0.713138492740816));
#10372=CARTESIAN_POINT('Ctrl Pts',(1.46055812562105,1.30629366210296,0.768258557763732));
#10373=CARTESIAN_POINT('Ctrl Pts',(1.44466308895875,1.3,0.797770130104052));
#10374=CARTESIAN_POINT('Ctrl Pts',(1.42894191624432,1.3,0.825000000000001));
#10375=CARTESIAN_POINT('',(0.59736109069228,1.55,0.0562114519197835));
#10376=CARTESIAN_POINT('',(0.125,1.55,-0.21650635094611));
#10377=CARTESIAN_POINT('Ctrl Pts',(0.59736109069228,1.55,0.0562114519197835));
#10378=CARTESIAN_POINT('Ctrl Pts',(0.59736109069228,1.58183602855499,0.0562114519197835));
#10379=CARTESIAN_POINT('Ctrl Pts',(0.596809586309859,1.61548166177648,0.0633319361811907));
#10380=CARTESIAN_POINT('Ctrl Pts',(0.593243052195919,1.67693412158597,0.0908585874761106));
#10381=CARTESIAN_POINT('Ctrl Pts',(0.590063593315144,1.70478184753241,0.111151766652641));
#10382=CARTESIAN_POINT('Ctrl Pts',(0.579820497891285,1.74874496453875,0.15600214762839));
#10383=CARTESIAN_POINT('Ctrl Pts',(0.572042315803119,1.76792916820474,0.183678633836535));
#10384=CARTESIAN_POINT('Ctrl Pts',(0.549947124580676,1.79356669468566,0.241926459727039));
#10385=CARTESIAN_POINT('Ctrl Pts',(0.53551402125728,1.8,0.27246250701687));
#10386=CARTESIAN_POINT('Ctrl Pts',(0.503716463284046,1.8,0.32753749298313));
#10387=CARTESIAN_POINT('Ctrl Pts',(0.484488022261586,1.79356669468566,0.355304950761552));
#10388=CARTESIAN_POINT('Ctrl Pts',(0.445091520936419,1.76792916820474,0.403563860606914));
#10389=CARTESIAN_POINT('Ctrl Pts',(0.425012071836758,1.74874496453875,0.4241382069946));
#10390=CARTESIAN_POINT('Ctrl Pts',(0.391292050254278,1.70478184753241,0.455434178332924));
#10391=CARTESIAN_POINT('Ctrl Pts',(0.375307371004241,1.67693412158597,0.468334260082228));
#10392=CARTESIAN_POINT('Ctrl Pts',(0.353251858758695,1.61548166177647,0.485186294875824));
#10393=CARTESIAN_POINT('Ctrl Pts',(0.347361090692279,1.58183602855499,0.489224153812003));
#10394=CARTESIAN_POINT('Ctrl Pts',(0.347361090692279,1.51816397144501,0.489224153812003));
#10395=CARTESIAN_POINT('Ctrl Pts',(0.353251858758695,1.48451833822352,0.485186294875824));
#10396=CARTESIAN_POINT('Ctrl Pts',(0.375307371004241,1.42306587841403,0.468334260082228));
#10397=CARTESIAN_POINT('Ctrl Pts',(0.391292050254278,1.39521815246759,0.455434178332924));
#10398=CARTESIAN_POINT('Ctrl Pts',(0.425012071836758,1.35125503546125,0.4241382069946));
#10399=CARTESIAN_POINT('Ctrl Pts',(0.445091520936418,1.33207083179526,0.403563860606914));
#10400=CARTESIAN_POINT('Ctrl Pts',(0.484488022261586,1.30643330531434,0.355304950761552));
#10401=CARTESIAN_POINT('Ctrl Pts',(0.503716463284046,1.3,0.32753749298313));
#10402=CARTESIAN_POINT('Ctrl Pts',(0.53551402125728,1.3,0.27246250701687));
#10403=CARTESIAN_POINT('Ctrl Pts',(0.549947124580676,1.30643330531434,0.241926459727039));
#10404=CARTESIAN_POINT('Ctrl Pts',(0.572042315803119,1.33207083179526,0.183678633836535));
#10405=CARTESIAN_POINT('Ctrl Pts',(0.579820497891285,1.35125503546125,0.15600214762839));
#10406=CARTESIAN_POINT('Ctrl Pts',(0.590063593315144,1.39521815246759,0.111151766652641));
#10407=CARTESIAN_POINT('Ctrl Pts',(0.593243052195919,1.42306587841403,0.0908585874761105));
#10408=CARTESIAN_POINT('Ctrl Pts',(0.596809586309859,1.48451833822352,0.0633319361811906));
#10409=CARTESIAN_POINT('Ctrl Pts',(0.59736109069228,1.51816397144501,0.0562114519197835));
#10410=CARTESIAN_POINT('Ctrl Pts',(0.59736109069228,1.55,0.0562114519197835));
#10411=CARTESIAN_POINT('Origin',(0.,1.55,0.));
#10412=CARTESIAN_POINT('',(-0.347361090692279,1.55,-0.489224153812003));
#10413=CARTESIAN_POINT('Ctrl Pts',(-0.347361090692279,1.55,-0.489224153812003));
#10414=CARTESIAN_POINT('Ctrl Pts',(-0.347361090692279,1.51816397144501,
-0.489224153812003));
#10415=CARTESIAN_POINT('Ctrl Pts',(-0.353251858758695,1.48451833822352,
-0.485186294875824));
#10416=CARTESIAN_POINT('Ctrl Pts',(-0.375307371004241,1.42306587841403,
-0.468334260082228));
#10417=CARTESIAN_POINT('Ctrl Pts',(-0.391292050254278,1.39521815246759,
-0.455434178332924));
#10418=CARTESIAN_POINT('Ctrl Pts',(-0.425012071836758,1.35125503546125,
-0.4241382069946));
#10419=CARTESIAN_POINT('Ctrl Pts',(-0.445091520936419,1.33207083179526,
-0.403563860606914));
#10420=CARTESIAN_POINT('Ctrl Pts',(-0.484488022261586,1.30643330531434,
-0.355304950761552));
#10421=CARTESIAN_POINT('Ctrl Pts',(-0.503716463284046,1.3,-0.32753749298313));
#10422=CARTESIAN_POINT('Ctrl Pts',(-0.53551402125728,1.3,-0.27246250701687));
#10423=CARTESIAN_POINT('Ctrl Pts',(-0.549947124580676,1.30643330531434,
-0.241926459727039));
#10424=CARTESIAN_POINT('Ctrl Pts',(-0.572042315803119,1.33207083179526,
-0.183678633836535));
#10425=CARTESIAN_POINT('Ctrl Pts',(-0.579820497891285,1.35125503546125,
-0.15600214762839));
#10426=CARTESIAN_POINT('Ctrl Pts',(-0.590063593315144,1.39521815246759,
-0.111151766652641));
#10427=CARTESIAN_POINT('Ctrl Pts',(-0.593243052195918,1.42306587841403,
-0.0908585874761106));
#10428=CARTESIAN_POINT('Ctrl Pts',(-0.596809586309859,1.48451833822352,
-0.0633319361811906));
#10429=CARTESIAN_POINT('Ctrl Pts',(-0.597361090692279,1.51816397144501,
-0.0562114519197835));
#10430=CARTESIAN_POINT('Ctrl Pts',(-0.597361090692279,1.58183602855499,
-0.0562114519197835));
#10431=CARTESIAN_POINT('Ctrl Pts',(-0.596809586309859,1.61548166177647,
-0.0633319361811905));
#10432=CARTESIAN_POINT('Ctrl Pts',(-0.593243052195918,1.67693412158597,
-0.0908585874761104));
#10433=CARTESIAN_POINT('Ctrl Pts',(-0.590063593315144,1.70478184753241,
-0.111151766652641));
#10434=CARTESIAN_POINT('Ctrl Pts',(-0.579820497891285,1.74874496453875,
-0.15600214762839));
#10435=CARTESIAN_POINT('Ctrl Pts',(-0.572042315803118,1.76792916820474,
-0.183678633836535));
#10436=CARTESIAN_POINT('Ctrl Pts',(-0.549947124580676,1.79356669468566,
-0.241926459727039));
#10437=CARTESIAN_POINT('Ctrl Pts',(-0.53551402125728,1.8,-0.27246250701687));
#10438=CARTESIAN_POINT('Ctrl Pts',(-0.503716463284046,1.8,-0.32753749298313));
#10439=CARTESIAN_POINT('Ctrl Pts',(-0.484488022261586,1.79356669468566,
-0.355304950761552));
#10440=CARTESIAN_POINT('Ctrl Pts',(-0.445091520936419,1.76792916820474,
-0.403563860606914));
#10441=CARTESIAN_POINT('Ctrl Pts',(-0.425012071836758,1.74874496453875,
-0.4241382069946));
#10442=CARTESIAN_POINT('Ctrl Pts',(-0.391292050254278,1.70478184753241,
-0.455434178332924));
#10443=CARTESIAN_POINT('Ctrl Pts',(-0.375307371004241,1.67693412158597,
-0.468334260082228));
#10444=CARTESIAN_POINT('Ctrl Pts',(-0.353251858758695,1.61548166177648,
-0.485186294875824));
#10445=CARTESIAN_POINT('Ctrl Pts',(-0.347361090692279,1.58183602855499,
-0.489224153812003));
#10446=CARTESIAN_POINT('Ctrl Pts',(-0.347361090692279,1.55,-0.489224153812003));
#10447=CARTESIAN_POINT('',(-1.28744468918255,1.55,-1.03198167246111));
#10448=CARTESIAN_POINT('',(0.125,1.55,-0.21650635094611));
#10449=CARTESIAN_POINT('',(-1.42894191624432,1.3,-0.825000000000001));
#10450=CARTESIAN_POINT('Ctrl Pts',(-1.42894191624432,1.3,-0.825000000000001));
#10451=CARTESIAN_POINT('Ctrl Pts',(-1.4132207435299,1.3,-0.852229869895949));
#10452=CARTESIAN_POINT('Ctrl Pts',(-1.39561049050871,1.30629366210296,-0.880751161609749));
#10453=CARTESIAN_POINT('Ctrl Pts',(-1.36172049302549,1.33182222741682,-0.932292094146256));
#10454=CARTESIAN_POINT('Ctrl Pts',(-1.34548213209931,1.35105447038507,-0.955340251466735));
#10455=CARTESIAN_POINT('Ctrl Pts',(-1.31917543061769,1.39539254159618,-0.991349264982991));
#10456=CARTESIAN_POINT('Ctrl Pts',(-1.30734972067592,1.42347183818157,-1.00672880483252));
#10457=CARTESIAN_POINT('Ctrl Pts',(-1.29146042158868,1.48505200040818,-1.02703269653942));
#10458=CARTESIAN_POINT('Ctrl Pts',(-1.28744468918255,1.51855708359447,-1.03198167246111));
#10459=CARTESIAN_POINT('Ctrl Pts',(-1.28744468918255,1.55,-1.03198167246111));
#10460=CARTESIAN_POINT('',(-1.42894191624432,1.8,-0.825000000000001));
#10461=CARTESIAN_POINT('Ctrl Pts',(-1.42894191624432,1.8,-0.825000000000001));
#10462=CARTESIAN_POINT('Ctrl Pts',(-1.44466308895875,1.8,-0.797770130104052));
#10463=CARTESIAN_POINT('Ctrl Pts',(-1.46055812562105,1.79370633789704,-0.768258557763732));
#10464=CARTESIAN_POINT('Ctrl Pts',(-1.48824888379079,1.76817777258318,-0.713138492740816));
#10465=CARTESIAN_POINT('Ctrl Pts',(-1.50008999307766,1.74894552961493,-0.687551581002689));
#10466=CARTESIAN_POINT('Ctrl Pts',(-1.51812136280714,1.70460745840382,-0.646764802471699));
#10467=CARTESIAN_POINT('Ctrl Pts',(-1.52552758004446,1.67652816181843,-0.628833667319578));
#10468=CARTESIAN_POINT('Ctrl Pts',(-1.53516661651472,1.61494799959182,-0.60492118480825));
#10469=CARTESIAN_POINT('Ctrl Pts',(-1.53744468918255,1.58144291640553,-0.598968970568896));
#10470=CARTESIAN_POINT('Ctrl Pts',(-1.53744468918255,1.51855708359447,-0.598968970568896));
#10471=CARTESIAN_POINT('Ctrl Pts',(-1.53516661651472,1.48505200040818,-0.60492118480825));
#10472=CARTESIAN_POINT('Ctrl Pts',(-1.52552758004446,1.42347183818157,-0.628833667319578));
#10473=CARTESIAN_POINT('Ctrl Pts',(-1.51812136280714,1.39539254159618,-0.646764802471699));
#10474=CARTESIAN_POINT('Ctrl Pts',(-1.50008999307766,1.35105447038507,-0.687551581002689));
#10475=CARTESIAN_POINT('Ctrl Pts',(-1.48824888379079,1.33182222741682,-0.713138492740816));
#10476=CARTESIAN_POINT('Ctrl Pts',(-1.46055812562105,1.30629366210296,-0.768258557763732));
#10477=CARTESIAN_POINT('Ctrl Pts',(-1.44466308895875,1.3,-0.797770130104052));
#10478=CARTESIAN_POINT('Ctrl Pts',(-1.42894191624432,1.3,-0.825000000000001));
#10479=CARTESIAN_POINT('Ctrl Pts',(-1.28744468918255,1.55,-1.03198167246111));
#10480=CARTESIAN_POINT('Ctrl Pts',(-1.28744468918255,1.58144291640553,-1.03198167246111));
#10481=CARTESIAN_POINT('Ctrl Pts',(-1.29146042158868,1.61494799959182,-1.02703269653942));
#10482=CARTESIAN_POINT('Ctrl Pts',(-1.30734972067592,1.67652816181843,-1.00672880483252));
#10483=CARTESIAN_POINT('Ctrl Pts',(-1.31917543061769,1.70460745840382,-0.991349264982991));
#10484=CARTESIAN_POINT('Ctrl Pts',(-1.34548213209931,1.74894552961493,-0.955340251466734));
#10485=CARTESIAN_POINT('Ctrl Pts',(-1.36172049302549,1.76817777258318,-0.932292094146256));
#10486=CARTESIAN_POINT('Ctrl Pts',(-1.39561049050871,1.79370633789704,-0.880751161609749));
#10487=CARTESIAN_POINT('Ctrl Pts',(-1.4132207435299,1.8,-0.852229869895949));
#10488=CARTESIAN_POINT('Ctrl Pts',(-1.42894191624432,1.8,-0.825000000000001));
#10489=CARTESIAN_POINT('Origin',(0.,1.55,0.));
#10490=CARTESIAN_POINT('',(-1.65,0.85,-2.02066721859313E-16));
#10491=CARTESIAN_POINT('Origin',(0.,0.85,0.));
#10492=CARTESIAN_POINT('',(-1.65,2.25,-2.02066721859313E-16));
#10493=CARTESIAN_POINT('',(-1.65,1.55,-2.02066721859313E-16));
#10494=CARTESIAN_POINT('Origin',(0.,2.25,0.));
#10495=CARTESIAN_POINT('',(-1.42894191624432,1.3,0.825));
#10496=CARTESIAN_POINT('',(-1.42894191624432,1.8,0.825));
#10497=CARTESIAN_POINT('Ctrl Pts',(-1.42894191624432,1.3,0.825));
#10498=CARTESIAN_POINT('Ctrl Pts',(-1.44466308895875,1.3,0.797770130104051));
#10499=CARTESIAN_POINT('Ctrl Pts',(-1.46055812562105,1.30629366210296,0.768258557763731));
#10500=CARTESIAN_POINT('Ctrl Pts',(-1.48824888379079,1.33182222741682,0.713138492740815));
#10501=CARTESIAN_POINT('Ctrl Pts',(-1.50008999307766,1.35105447038507,0.687551581002688));
#10502=CARTESIAN_POINT('Ctrl Pts',(-1.51812136280714,1.39539254159618,0.646764802471698));
#10503=CARTESIAN_POINT('Ctrl Pts',(-1.52552758004446,1.42347183818157,0.628833667319577));
#10504=CARTESIAN_POINT('Ctrl Pts',(-1.53516661651472,1.48505200040818,0.604921184808249));
#10505=CARTESIAN_POINT('Ctrl Pts',(-1.53744468918255,1.51855708359447,0.598968970568895));
#10506=CARTESIAN_POINT('Ctrl Pts',(-1.53744468918255,1.58144291640553,0.598968970568895));
#10507=CARTESIAN_POINT('Ctrl Pts',(-1.53516661651472,1.61494799959182,0.604921184808249));
#10508=CARTESIAN_POINT('Ctrl Pts',(-1.52552758004446,1.67652816181843,0.628833667319577));
#10509=CARTESIAN_POINT('Ctrl Pts',(-1.51812136280714,1.70460745840382,0.646764802471698));
#10510=CARTESIAN_POINT('Ctrl Pts',(-1.50008999307766,1.74894552961493,0.687551581002688));
#10511=CARTESIAN_POINT('Ctrl Pts',(-1.48824888379079,1.76817777258318,0.713138492740815));
#10512=CARTESIAN_POINT('Ctrl Pts',(-1.46055812562105,1.79370633789704,0.768258557763731));
#10513=CARTESIAN_POINT('Ctrl Pts',(-1.44466308895875,1.8,0.797770130104051));
#10514=CARTESIAN_POINT('Ctrl Pts',(-1.42894191624432,1.8,0.825));
#10515=CARTESIAN_POINT('',(-1.28744468918255,1.55,1.03198167246111));
#10516=CARTESIAN_POINT('Ctrl Pts',(-1.42894191624432,1.8,0.825));
#10517=CARTESIAN_POINT('Ctrl Pts',(-1.4132207435299,1.8,0.852229869895948));
#10518=CARTESIAN_POINT('Ctrl Pts',(-1.39561049050871,1.79370633789704,0.880751161609747));
#10519=CARTESIAN_POINT('Ctrl Pts',(-1.36172049302549,1.76817777258318,0.932292094146255));
#10520=CARTESIAN_POINT('Ctrl Pts',(-1.34548213209931,1.74894552961493,0.955340251466733));
#10521=CARTESIAN_POINT('Ctrl Pts',(-1.31917543061769,1.70460745840382,0.991349264982989));
#10522=CARTESIAN_POINT('Ctrl Pts',(-1.30734972067592,1.67652816181843,1.00672880483252));
#10523=CARTESIAN_POINT('Ctrl Pts',(-1.29146042158868,1.61494799959182,1.02703269653942));
#10524=CARTESIAN_POINT('Ctrl Pts',(-1.28744468918255,1.58144291640553,1.03198167246111));
#10525=CARTESIAN_POINT('Ctrl Pts',(-1.28744468918255,1.55,1.03198167246111));
#10526=CARTESIAN_POINT('Ctrl Pts',(-1.28744468918255,1.55,1.03198167246111));
#10527=CARTESIAN_POINT('Ctrl Pts',(-1.28744468918255,1.51855708359447,1.03198167246111));
#10528=CARTESIAN_POINT('Ctrl Pts',(-1.29146042158868,1.48505200040818,1.02703269653942));
#10529=CARTESIAN_POINT('Ctrl Pts',(-1.30734972067592,1.42347183818157,1.00672880483252));
#10530=CARTESIAN_POINT('Ctrl Pts',(-1.31917543061769,1.39539254159618,0.99134926498299));
#10531=CARTESIAN_POINT('Ctrl Pts',(-1.34548213209931,1.35105447038508,0.955340251466733));
#10532=CARTESIAN_POINT('Ctrl Pts',(-1.36172049302549,1.33182222741682,0.932292094146255));
#10533=CARTESIAN_POINT('Ctrl Pts',(-1.39561049050871,1.30629366210296,0.880751161609748));
#10534=CARTESIAN_POINT('Ctrl Pts',(-1.4132207435299,1.3,0.852229869895949));
#10535=CARTESIAN_POINT('Ctrl Pts',(-1.42894191624432,1.3,0.825));
#10536=CARTESIAN_POINT('',(1.42894191624432,1.8,-0.825));
#10537=CARTESIAN_POINT('',(1.42894191624432,1.3,-0.825));
#10538=CARTESIAN_POINT('Ctrl Pts',(1.42894191624432,1.8,-0.825));
#10539=CARTESIAN_POINT('Ctrl Pts',(1.4132207435299,1.8,-0.852229869895949));
#10540=CARTESIAN_POINT('Ctrl Pts',(1.39561049050871,1.79370633789704,-0.880751161609748));
#10541=CARTESIAN_POINT('Ctrl Pts',(1.36172049302549,1.76817777258318,-0.932292094146255));
#10542=CARTESIAN_POINT('Ctrl Pts',(1.34548213209931,1.74894552961493,-0.955340251466734));
#10543=CARTESIAN_POINT('Ctrl Pts',(1.31917543061769,1.70460745840382,-0.99134926498299));
#10544=CARTESIAN_POINT('Ctrl Pts',(1.30734972067592,1.67652816181843,-1.00672880483252));
#10545=CARTESIAN_POINT('Ctrl Pts',(1.29146042158868,1.61494799959182,-1.02703269653942));
#10546=CARTESIAN_POINT('Ctrl Pts',(1.28744468918255,1.58144291640553,-1.03198167246111));
#10547=CARTESIAN_POINT('Ctrl Pts',(1.28744468918255,1.51855708359447,-1.03198167246111));
#10548=CARTESIAN_POINT('Ctrl Pts',(1.29146042158868,1.48505200040818,-1.02703269653942));
#10549=CARTESIAN_POINT('Ctrl Pts',(1.30734972067592,1.42347183818157,-1.00672880483252));
#10550=CARTESIAN_POINT('Ctrl Pts',(1.31917543061769,1.39539254159618,-0.99134926498299));
#10551=CARTESIAN_POINT('Ctrl Pts',(1.34548213209931,1.35105447038507,-0.955340251466734));
#10552=CARTESIAN_POINT('Ctrl Pts',(1.36172049302549,1.33182222741682,-0.932292094146255));
#10553=CARTESIAN_POINT('Ctrl Pts',(1.39561049050871,1.30629366210296,-0.880751161609748));
#10554=CARTESIAN_POINT('Ctrl Pts',(1.4132207435299,1.3,-0.852229869895948));
#10555=CARTESIAN_POINT('Ctrl Pts',(1.42894191624432,1.3,-0.825));
#10556=CARTESIAN_POINT('',(1.53744468918255,1.55,-0.598968970568895));
#10557=CARTESIAN_POINT('Ctrl Pts',(1.42894191624432,1.3,-0.825));
#10558=CARTESIAN_POINT('Ctrl Pts',(1.44466308895875,1.3,-0.797770130104051));
#10559=CARTESIAN_POINT('Ctrl Pts',(1.46055812562105,1.30629366210296,-0.768258557763731));
#10560=CARTESIAN_POINT('Ctrl Pts',(1.48824888379079,1.33182222741682,-0.713138492740815));
#10561=CARTESIAN_POINT('Ctrl Pts',(1.50008999307766,1.35105447038507,-0.687551581002688));
#10562=CARTESIAN_POINT('Ctrl Pts',(1.51812136280714,1.39539254159618,-0.646764802471698));
#10563=CARTESIAN_POINT('Ctrl Pts',(1.52552758004446,1.42347183818157,-0.628833667319577));
#10564=CARTESIAN_POINT('Ctrl Pts',(1.53516661651472,1.48505200040818,-0.604921184808249));
#10565=CARTESIAN_POINT('Ctrl Pts',(1.53744468918255,1.51855708359447,-0.598968970568895));
#10566=CARTESIAN_POINT('Ctrl Pts',(1.53744468918255,1.55,-0.598968970568895));
#10567=CARTESIAN_POINT('Ctrl Pts',(1.53744468918255,1.55,-0.598968970568895));
#10568=CARTESIAN_POINT('Ctrl Pts',(1.53744468918255,1.58144291640553,-0.598968970568895));
#10569=CARTESIAN_POINT('Ctrl Pts',(1.53516661651472,1.61494799959182,-0.604921184808249));
#10570=CARTESIAN_POINT('Ctrl Pts',(1.52552758004446,1.67652816181843,-0.628833667319577));
#10571=CARTESIAN_POINT('Ctrl Pts',(1.51812136280714,1.70460745840382,-0.646764802471698));
#10572=CARTESIAN_POINT('Ctrl Pts',(1.50008999307766,1.74894552961493,-0.687551581002688));
#10573=CARTESIAN_POINT('Ctrl Pts',(1.48824888379079,1.76817777258318,-0.713138492740815));
#10574=CARTESIAN_POINT('Ctrl Pts',(1.46055812562105,1.79370633789704,-0.768258557763731));
#10575=CARTESIAN_POINT('Ctrl Pts',(1.44466308895875,1.8,-0.797770130104051));
#10576=CARTESIAN_POINT('Ctrl Pts',(1.42894191624432,1.8,-0.825));
#10577=CARTESIAN_POINT('',(0.,1.3,-1.65));
#10578=CARTESIAN_POINT('',(0.,1.8,-1.65));
#10579=CARTESIAN_POINT('Ctrl Pts',(1.38777878078145E-17,1.3,-1.65));
#10580=CARTESIAN_POINT('Ctrl Pts',(0.0314423454288489,1.3,-1.65));
#10581=CARTESIAN_POINT('Ctrl Pts',(0.0649476351123396,1.30629366210296,
-1.64900971937348));
#10582=CARTESIAN_POINT('Ctrl Pts',(0.126528390765307,1.33182222741682,-1.64543058688707));
#10583=CARTESIAN_POINT('Ctrl Pts',(0.154607860978348,1.35105447038507,-1.64289183246942));
#10584=CARTESIAN_POINT('Ctrl Pts',(0.198945932189457,1.39539254159618,-1.63811406745469));
#10585=CARTESIAN_POINT('Ctrl Pts',(0.218177859368546,1.42347183818157,-1.63556247215209));
#10586=CARTESIAN_POINT('Ctrl Pts',(0.243706194926033,1.48505200040818,-1.63195388134767));
#10587=CARTESIAN_POINT('Ctrl Pts',(0.25,1.51855708359447,-1.63095064303001));
#10588=CARTESIAN_POINT('Ctrl Pts',(0.25,1.58144291640553,-1.63095064303001));
#10589=CARTESIAN_POINT('Ctrl Pts',(0.243706194926033,1.61494799959182,-1.63195388134767));
#10590=CARTESIAN_POINT('Ctrl Pts',(0.218177859368546,1.67652816181843,-1.63556247215209));
#10591=CARTESIAN_POINT('Ctrl Pts',(0.198945932189457,1.70460745840382,-1.63811406745469));
#10592=CARTESIAN_POINT('Ctrl Pts',(0.154607860978349,1.74894552961493,-1.64289183246942));
#10593=CARTESIAN_POINT('Ctrl Pts',(0.126528390765307,1.76817777258318,-1.64543058688707));
#10594=CARTESIAN_POINT('Ctrl Pts',(0.0649476351123398,1.79370633789704,
-1.64900971937348));
#10595=CARTESIAN_POINT('Ctrl Pts',(0.031442345428849,1.8,-1.65));
#10596=CARTESIAN_POINT('Ctrl Pts',(7.63278329429795E-17,1.8,-1.65));
#10597=CARTESIAN_POINT('',(-0.25,1.55,-1.63095064303001));
#10598=CARTESIAN_POINT('Ctrl Pts',(9.0205620750794E-17,1.8,-1.65));
#10599=CARTESIAN_POINT('Ctrl Pts',(-0.0314423454288488,1.8,-1.65));
#10600=CARTESIAN_POINT('Ctrl Pts',(-0.0649476351123396,1.79370633789704,
-1.64900971937348));
#10601=CARTESIAN_POINT('Ctrl Pts',(-0.126528390765307,1.76817777258318,
-1.64543058688707));
#10602=CARTESIAN_POINT('Ctrl Pts',(-0.154607860978348,1.74894552961493,
-1.64289183246942));
#10603=CARTESIAN_POINT('Ctrl Pts',(-0.198945932189456,1.70460745840382,
-1.63811406745469));
#10604=CARTESIAN_POINT('Ctrl Pts',(-0.218177859368546,1.67652816181843,
-1.63556247215209));
#10605=CARTESIAN_POINT('Ctrl Pts',(-0.243706194926033,1.61494799959182,
-1.63195388134767));
#10606=CARTESIAN_POINT('Ctrl Pts',(-0.25,1.58144291640553,-1.63095064303001));
#10607=CARTESIAN_POINT('Ctrl Pts',(-0.25,1.55,-1.63095064303001));
#10608=CARTESIAN_POINT('Ctrl Pts',(-0.25,1.55,-1.63095064303001));
#10609=CARTESIAN_POINT('Ctrl Pts',(-0.25,1.51855708359447,-1.63095064303001));
#10610=CARTESIAN_POINT('Ctrl Pts',(-0.243706194926033,1.48505200040818,
-1.63195388134767));
#10611=CARTESIAN_POINT('Ctrl Pts',(-0.218177859368546,1.42347183818157,
-1.63556247215209));
#10612=CARTESIAN_POINT('Ctrl Pts',(-0.198945932189457,1.39539254159618,
-1.63811406745469));
#10613=CARTESIAN_POINT('Ctrl Pts',(-0.154607860978349,1.35105447038507,
-1.64289183246942));
#10614=CARTESIAN_POINT('Ctrl Pts',(-0.126528390765307,1.33182222741682,
-1.64543058688707));
#10615=CARTESIAN_POINT('Ctrl Pts',(-0.0649476351123398,1.30629366210296,
-1.64900971937348));
#10616=CARTESIAN_POINT('Ctrl Pts',(-0.031442345428849,1.3,-1.65));
#10617=CARTESIAN_POINT('Ctrl Pts',(-4.85722573273506E-17,1.3,-1.65));
#10618=CARTESIAN_POINT('',(0.,1.8,1.65));
#10619=CARTESIAN_POINT('',(0.,1.3,1.65));
#10620=CARTESIAN_POINT('Ctrl Pts',(8.32667268468867E-17,1.8,1.65));
#10621=CARTESIAN_POINT('Ctrl Pts',(0.031442345428849,1.8,1.65));
#10622=CARTESIAN_POINT('Ctrl Pts',(0.0649476351123398,1.79370633789704,
1.64900971937348));
#10623=CARTESIAN_POINT('Ctrl Pts',(0.126528390765307,1.76817777258318,1.64543058688707));
#10624=CARTESIAN_POINT('Ctrl Pts',(0.154607860978349,1.74894552961493,1.64289183246942));
#10625=CARTESIAN_POINT('Ctrl Pts',(0.198945932189457,1.70460745840382,1.63811406745469));
#10626=CARTESIAN_POINT('Ctrl Pts',(0.218177859368546,1.67652816181843,1.63556247215209));
#10627=CARTESIAN_POINT('Ctrl Pts',(0.243706194926033,1.61494799959182,1.63195388134767));
#10628=CARTESIAN_POINT('Ctrl Pts',(0.25,1.58144291640553,1.63095064303001));
#10629=CARTESIAN_POINT('Ctrl Pts',(0.25,1.51855708359447,1.63095064303001));
#10630=CARTESIAN_POINT('Ctrl Pts',(0.243706194926033,1.48505200040818,1.63195388134767));
#10631=CARTESIAN_POINT('Ctrl Pts',(0.218177859368546,1.42347183818157,1.63556247215209));
#10632=CARTESIAN_POINT('Ctrl Pts',(0.198945932189457,1.39539254159618,1.63811406745469));
#10633=CARTESIAN_POINT('Ctrl Pts',(0.154607860978348,1.35105447038507,1.64289183246942));
#10634=CARTESIAN_POINT('Ctrl Pts',(0.126528390765307,1.33182222741682,1.64543058688707));
#10635=CARTESIAN_POINT('Ctrl Pts',(0.0649476351123397,1.30629366210296,
1.64900971937348));
#10636=CARTESIAN_POINT('Ctrl Pts',(0.0314423454288488,1.3,1.65));
#10637=CARTESIAN_POINT('Ctrl Pts',(-1.38777878078145E-17,1.3,1.65));
#10638=CARTESIAN_POINT('',(-0.25,1.55,1.63095064303001));
#10639=CARTESIAN_POINT('Ctrl Pts',(-5.55111512312578E-17,1.3,1.65));
#10640=CARTESIAN_POINT('Ctrl Pts',(-0.031442345428849,1.3,1.65));
#10641=CARTESIAN_POINT('Ctrl Pts',(-0.0649476351123398,1.30629366210296,
1.64900971937348));
#10642=CARTESIAN_POINT('Ctrl Pts',(-0.126528390765307,1.33182222741682,
1.64543058688707));
#10643=CARTESIAN_POINT('Ctrl Pts',(-0.154607860978349,1.35105447038507,
1.64289183246942));
#10644=CARTESIAN_POINT('Ctrl Pts',(-0.198945932189457,1.39539254159618,
1.63811406745469));
#10645=CARTESIAN_POINT('Ctrl Pts',(-0.218177859368546,1.42347183818157,
1.63556247215209));
#10646=CARTESIAN_POINT('Ctrl Pts',(-0.243706194926033,1.48505200040818,
1.63195388134767));
#10647=CARTESIAN_POINT('Ctrl Pts',(-0.25,1.51855708359447,1.63095064303001));
#10648=CARTESIAN_POINT('Ctrl Pts',(-0.25,1.55,1.63095064303001));
#10649=CARTESIAN_POINT('Ctrl Pts',(-0.25,1.55,1.63095064303001));
#10650=CARTESIAN_POINT('Ctrl Pts',(-0.25,1.58144291640553,1.63095064303001));
#10651=CARTESIAN_POINT('Ctrl Pts',(-0.243706194926033,1.61494799959182,
1.63195388134767));
#10652=CARTESIAN_POINT('Ctrl Pts',(-0.218177859368546,1.67652816181843,
1.63556247215209));
#10653=CARTESIAN_POINT('Ctrl Pts',(-0.198945932189456,1.70460745840382,
1.63811406745469));
#10654=CARTESIAN_POINT('Ctrl Pts',(-0.154607860978348,1.74894552961493,
1.64289183246942));
#10655=CARTESIAN_POINT('Ctrl Pts',(-0.126528390765307,1.76817777258318,
1.64543058688707));
#10656=CARTESIAN_POINT('Ctrl Pts',(-0.0649476351123396,1.79370633789704,
1.64900971937348));
#10657=CARTESIAN_POINT('Ctrl Pts',(-0.0314423454288488,1.8,1.65));
#10658=CARTESIAN_POINT('Ctrl Pts',(7.63278329429795E-17,1.8,1.65));
#10659=CARTESIAN_POINT('Origin',(0.,1.55,0.));
#10660=CARTESIAN_POINT('',(-0.34736109069228,1.55,0.489224153812002));
#10661=CARTESIAN_POINT('',(0.125,1.55,0.21650635094611));
#10662=CARTESIAN_POINT('Ctrl Pts',(-0.34736109069228,1.55,0.489224153812002));
#10663=CARTESIAN_POINT('Ctrl Pts',(-0.34736109069228,1.58183602855499,0.489224153812002));
#10664=CARTESIAN_POINT('Ctrl Pts',(-0.353251858758695,1.61548166177648,
0.485186294875824));
#10665=CARTESIAN_POINT('Ctrl Pts',(-0.375307371004242,1.67693412158597,
0.468334260082228));
#10666=CARTESIAN_POINT('Ctrl Pts',(-0.391292050254279,1.70478184753241,
0.455434178332924));
#10667=CARTESIAN_POINT('Ctrl Pts',(-0.425012071836758,1.74874496453875,
0.424138206994599));
#10668=CARTESIAN_POINT('Ctrl Pts',(-0.445091520936419,1.76792916820474,
0.403563860606914));
#10669=CARTESIAN_POINT('Ctrl Pts',(-0.484488022261587,1.79356669468566,
0.355304950761552));
#10670=CARTESIAN_POINT('Ctrl Pts',(-0.503716463284046,1.8,0.32753749298313));
#10671=CARTESIAN_POINT('Ctrl Pts',(-0.535514021257281,1.8,0.27246250701687));
#10672=CARTESIAN_POINT('Ctrl Pts',(-0.549947124580677,1.79356669468566,
0.241926459727038));
#10673=CARTESIAN_POINT('Ctrl Pts',(-0.572042315803119,1.76792916820474,
0.183678633836535));
#10674=CARTESIAN_POINT('Ctrl Pts',(-0.579820497891285,1.74874496453875,
0.156002147628389));
#10675=CARTESIAN_POINT('Ctrl Pts',(-0.590063593315144,1.70478184753241,
0.11115176665264));
#10676=CARTESIAN_POINT('Ctrl Pts',(-0.593243052195919,1.67693412158597,
0.0908585874761102));
#10677=CARTESIAN_POINT('Ctrl Pts',(-0.596809586309859,1.61548166177648,
0.0633319361811903));
#10678=CARTESIAN_POINT('Ctrl Pts',(-0.59736109069228,1.58183602855499,0.0562114519197831));
#10679=CARTESIAN_POINT('Ctrl Pts',(-0.59736109069228,1.51816397144501,0.0562114519197831));
#10680=CARTESIAN_POINT('Ctrl Pts',(-0.596809586309859,1.48451833822352,
0.0633319361811902));
#10681=CARTESIAN_POINT('Ctrl Pts',(-0.593243052195919,1.42306587841403,
0.0908585874761101));
#10682=CARTESIAN_POINT('Ctrl Pts',(-0.590063593315144,1.39521815246759,
0.11115176665264));
#10683=CARTESIAN_POINT('Ctrl Pts',(-0.579820497891285,1.35125503546125,
0.156002147628389));
#10684=CARTESIAN_POINT('Ctrl Pts',(-0.572042315803119,1.33207083179526,
0.183678633836535));
#10685=CARTESIAN_POINT('Ctrl Pts',(-0.549947124580676,1.30643330531434,
0.241926459727038));
#10686=CARTESIAN_POINT('Ctrl Pts',(-0.535514021257281,1.3,0.27246250701687));
#10687=CARTESIAN_POINT('Ctrl Pts',(-0.503716463284046,1.3,0.32753749298313));
#10688=CARTESIAN_POINT('Ctrl Pts',(-0.484488022261587,1.30643330531434,
0.355304950761552));
#10689=CARTESIAN_POINT('Ctrl Pts',(-0.445091520936419,1.33207083179526,
0.403563860606914));
#10690=CARTESIAN_POINT('Ctrl Pts',(-0.425012071836758,1.35125503546125,
0.424138206994599));
#10691=CARTESIAN_POINT('Ctrl Pts',(-0.391292050254279,1.39521815246759,
0.455434178332924));
#10692=CARTESIAN_POINT('Ctrl Pts',(-0.375307371004241,1.42306587841403,
0.468334260082228));
#10693=CARTESIAN_POINT('Ctrl Pts',(-0.353251858758695,1.48451833822352,
0.485186294875824));
#10694=CARTESIAN_POINT('Ctrl Pts',(-0.34736109069228,1.51816397144501,0.489224153812002));
#10695=CARTESIAN_POINT('Ctrl Pts',(-0.34736109069228,1.55,0.489224153812002));
#10696=CARTESIAN_POINT('Origin',(0.,1.55,0.));
#10697=CARTESIAN_POINT('',(0.59736109069228,1.55,-0.0562114519197831));
#10698=CARTESIAN_POINT('Ctrl Pts',(0.59736109069228,1.55,-0.0562114519197831));
#10699=CARTESIAN_POINT('Ctrl Pts',(0.59736109069228,1.51816397144501,-0.0562114519197831));
#10700=CARTESIAN_POINT('Ctrl Pts',(0.596809586309859,1.48451833822352,-0.0633319361811902));
#10701=CARTESIAN_POINT('Ctrl Pts',(0.593243052195919,1.42306587841403,-0.0908585874761101));
#10702=CARTESIAN_POINT('Ctrl Pts',(0.590063593315144,1.39521815246759,-0.11115176665264));
#10703=CARTESIAN_POINT('Ctrl Pts',(0.579820497891285,1.35125503546125,-0.156002147628389));
#10704=CARTESIAN_POINT('Ctrl Pts',(0.572042315803119,1.33207083179526,-0.183678633836535));
#10705=CARTESIAN_POINT('Ctrl Pts',(0.549947124580677,1.30643330531434,-0.241926459727038));
#10706=CARTESIAN_POINT('Ctrl Pts',(0.535514021257281,1.3,-0.27246250701687));
#10707=CARTESIAN_POINT('Ctrl Pts',(0.503716463284046,1.3,-0.32753749298313));
#10708=CARTESIAN_POINT('Ctrl Pts',(0.484488022261587,1.30643330531434,-0.355304950761552));
#10709=CARTESIAN_POINT('Ctrl Pts',(0.445091520936419,1.33207083179526,-0.403563860606914));
#10710=CARTESIAN_POINT('Ctrl Pts',(0.425012071836758,1.35125503546125,-0.424138206994599));
#10711=CARTESIAN_POINT('Ctrl Pts',(0.391292050254279,1.39521815246759,-0.455434178332924));
#10712=CARTESIAN_POINT('Ctrl Pts',(0.375307371004241,1.42306587841403,-0.468334260082228));
#10713=CARTESIAN_POINT('Ctrl Pts',(0.353251858758695,1.48451833822352,-0.485186294875824));
#10714=CARTESIAN_POINT('Ctrl Pts',(0.34736109069228,1.51816397144501,-0.489224153812002));
#10715=CARTESIAN_POINT('Ctrl Pts',(0.34736109069228,1.58183602855499,-0.489224153812002));
#10716=CARTESIAN_POINT('Ctrl Pts',(0.353251858758695,1.61548166177647,-0.485186294875824));
#10717=CARTESIAN_POINT('Ctrl Pts',(0.375307371004241,1.67693412158597,-0.468334260082228));
#10718=CARTESIAN_POINT('Ctrl Pts',(0.391292050254279,1.70478184753241,-0.455434178332924));
#10719=CARTESIAN_POINT('Ctrl Pts',(0.425012071836758,1.74874496453875,-0.424138206994599));
#10720=CARTESIAN_POINT('Ctrl Pts',(0.445091520936419,1.76792916820474,-0.403563860606914));
#10721=CARTESIAN_POINT('Ctrl Pts',(0.484488022261587,1.79356669468566,-0.355304950761552));
#10722=CARTESIAN_POINT('Ctrl Pts',(0.503716463284046,1.8,-0.32753749298313));
#10723=CARTESIAN_POINT('Ctrl Pts',(0.535514021257281,1.8,-0.27246250701687));
#10724=CARTESIAN_POINT('Ctrl Pts',(0.549947124580677,1.79356669468566,-0.241926459727038));
#10725=CARTESIAN_POINT('Ctrl Pts',(0.572042315803119,1.76792916820474,-0.183678633836535));
#10726=CARTESIAN_POINT('Ctrl Pts',(0.579820497891285,1.74874496453875,-0.156002147628389));
#10727=CARTESIAN_POINT('Ctrl Pts',(0.590063593315144,1.70478184753241,-0.111151766652641));
#10728=CARTESIAN_POINT('Ctrl Pts',(0.593243052195919,1.67693412158597,-0.0908585874761104));
#10729=CARTESIAN_POINT('Ctrl Pts',(0.596809586309859,1.61548166177648,-0.0633319361811903));
#10730=CARTESIAN_POINT('Ctrl Pts',(0.59736109069228,1.58183602855499,-0.0562114519197831));
#10731=CARTESIAN_POINT('Ctrl Pts',(0.59736109069228,1.55,-0.0562114519197831));
#10732=CARTESIAN_POINT('',(0.125,1.55,0.21650635094611));
#10733=CARTESIAN_POINT('Origin',(0.,1.55,0.));
#10734=CARTESIAN_POINT('',(-0.25,1.55,-0.545435605731786));
#10735=CARTESIAN_POINT('',(-0.25,1.55,0.));
#10736=CARTESIAN_POINT('Ctrl Pts',(-0.25,1.55,-0.545435605731786));
#10737=CARTESIAN_POINT('Ctrl Pts',(-0.25,1.58183602855499,-0.545435605731786));
#10738=CARTESIAN_POINT('Ctrl Pts',(-0.243557727551164,1.61548166177648,
-0.548518231057014));
#10739=CARTESIAN_POINT('Ctrl Pts',(-0.217935681191677,1.67693412158597,
-0.559192847558338));
#10740=CARTESIAN_POINT('Ctrl Pts',(-0.198771543060865,1.70478184753241,
-0.566585944985565));
#10741=CARTESIAN_POINT('Ctrl Pts',(-0.154808426054527,1.74874496453875,
-0.580140354622989));
#10742=CARTESIAN_POINT('Ctrl Pts',(-0.1269507948667,1.76792916820474,-0.587242494443449));
#10743=CARTESIAN_POINT('Ctrl Pts',(-0.0654591023190899,1.79356669468566,
-0.597231410488591));
#10744=CARTESIAN_POINT('Ctrl Pts',(-0.0317975579732349,1.8,-0.6));
#10745=CARTESIAN_POINT('Ctrl Pts',(0.0317975579732349,1.8,-0.6));
#10746=CARTESIAN_POINT('Ctrl Pts',(0.0654591023190898,1.79356669468566,
-0.597231410488591));
#10747=CARTESIAN_POINT('Ctrl Pts',(0.1269507948667,1.76792916820474,-0.587242494443449));
#10748=CARTESIAN_POINT('Ctrl Pts',(0.154808426054527,1.74874496453875,-0.580140354622989));
#10749=CARTESIAN_POINT('Ctrl Pts',(0.198771543060865,1.70478184753241,-0.566585944985565));
#10750=CARTESIAN_POINT('Ctrl Pts',(0.217935681191677,1.67693412158597,-0.559192847558338));
#10751=CARTESIAN_POINT('Ctrl Pts',(0.243557727551164,1.61548166177648,-0.548518231057014));
#10752=CARTESIAN_POINT('Ctrl Pts',(0.25,1.58183602855499,-0.545435605731786));
#10753=CARTESIAN_POINT('Ctrl Pts',(0.25,1.51816397144501,-0.545435605731786));
#10754=CARTESIAN_POINT('Ctrl Pts',(0.243557727551164,1.48451833822352,-0.548518231057014));
#10755=CARTESIAN_POINT('Ctrl Pts',(0.217935681191677,1.42306587841403,-0.559192847558338));
#10756=CARTESIAN_POINT('Ctrl Pts',(0.198771543060865,1.39521815246759,-0.566585944985565));
#10757=CARTESIAN_POINT('Ctrl Pts',(0.154808426054527,1.35125503546125,-0.580140354622989));
#10758=CARTESIAN_POINT('Ctrl Pts',(0.1269507948667,1.33207083179526,-0.587242494443449));
#10759=CARTESIAN_POINT('Ctrl Pts',(0.0654591023190899,1.30643330531434,
-0.597231410488591));
#10760=CARTESIAN_POINT('Ctrl Pts',(0.0317975579732349,1.3,-0.6));
#10761=CARTESIAN_POINT('Ctrl Pts',(-0.0317975579732349,1.3,-0.6));
#10762=CARTESIAN_POINT('Ctrl Pts',(-0.0654591023190899,1.30643330531434,
-0.597231410488591));
#10763=CARTESIAN_POINT('Ctrl Pts',(-0.1269507948667,1.33207083179526,-0.587242494443449));
#10764=CARTESIAN_POINT('Ctrl Pts',(-0.154808426054527,1.35125503546125,
-0.580140354622989));
#10765=CARTESIAN_POINT('Ctrl Pts',(-0.198771543060865,1.39521815246759,
-0.566585944985565));
#10766=CARTESIAN_POINT('Ctrl Pts',(-0.217935681191677,1.42306587841403,
-0.559192847558338));
#10767=CARTESIAN_POINT('Ctrl Pts',(-0.243557727551164,1.48451833822352,
-0.548518231057014));
#10768=CARTESIAN_POINT('Ctrl Pts',(-0.25,1.51816397144501,-0.545435605731786));
#10769=CARTESIAN_POINT('Ctrl Pts',(-0.25,1.55,-0.545435605731786));
#10770=CARTESIAN_POINT('Origin',(0.,1.55,0.));
#10771=CARTESIAN_POINT('',(-0.25,1.55,0.545435605731786));
#10772=CARTESIAN_POINT('Ctrl Pts',(-0.25,1.55,0.545435605731786));
#10773=CARTESIAN_POINT('Ctrl Pts',(-0.25,1.51816397144501,0.545435605731786));
#10774=CARTESIAN_POINT('Ctrl Pts',(-0.243557727551164,1.48451833822352,
0.548518231057014));
#10775=CARTESIAN_POINT('Ctrl Pts',(-0.217935681191677,1.42306587841403,
0.559192847558338));
#10776=CARTESIAN_POINT('Ctrl Pts',(-0.198771543060865,1.39521815246759,
0.566585944985565));
#10777=CARTESIAN_POINT('Ctrl Pts',(-0.154808426054527,1.35125503546125,
0.580140354622989));
#10778=CARTESIAN_POINT('Ctrl Pts',(-0.1269507948667,1.33207083179526,0.587242494443449));
#10779=CARTESIAN_POINT('Ctrl Pts',(-0.0654591023190899,1.30643330531434,
0.597231410488591));
#10780=CARTESIAN_POINT('Ctrl Pts',(-0.0317975579732349,1.3,0.6));
#10781=CARTESIAN_POINT('Ctrl Pts',(0.0317975579732349,1.3,0.6));
#10782=CARTESIAN_POINT('Ctrl Pts',(0.0654591023190899,1.30643330531434,
0.597231410488591));
#10783=CARTESIAN_POINT('Ctrl Pts',(0.1269507948667,1.33207083179526,0.587242494443449));
#10784=CARTESIAN_POINT('Ctrl Pts',(0.154808426054527,1.35125503546125,0.580140354622989));
#10785=CARTESIAN_POINT('Ctrl Pts',(0.198771543060865,1.39521815246759,0.566585944985565));
#10786=CARTESIAN_POINT('Ctrl Pts',(0.217935681191677,1.42306587841403,0.559192847558338));
#10787=CARTESIAN_POINT('Ctrl Pts',(0.243557727551164,1.48451833822352,0.548518231057014));
#10788=CARTESIAN_POINT('Ctrl Pts',(0.25,1.51816397144501,0.545435605731786));
#10789=CARTESIAN_POINT('Ctrl Pts',(0.25,1.58183602855499,0.545435605731786));
#10790=CARTESIAN_POINT('Ctrl Pts',(0.243557727551164,1.61548166177648,0.548518231057014));
#10791=CARTESIAN_POINT('Ctrl Pts',(0.217935681191677,1.67693412158597,0.559192847558338));
#10792=CARTESIAN_POINT('Ctrl Pts',(0.198771543060865,1.70478184753241,0.566585944985565));
#10793=CARTESIAN_POINT('Ctrl Pts',(0.154808426054527,1.74874496453875,0.580140354622989));
#10794=CARTESIAN_POINT('Ctrl Pts',(0.1269507948667,1.76792916820474,0.587242494443449));
#10795=CARTESIAN_POINT('Ctrl Pts',(0.0654591023190898,1.79356669468566,
0.597231410488591));
#10796=CARTESIAN_POINT('Ctrl Pts',(0.0317975579732349,1.8,0.6));
#10797=CARTESIAN_POINT('Ctrl Pts',(-0.0317975579732349,1.8,0.6));
#10798=CARTESIAN_POINT('Ctrl Pts',(-0.0654591023190898,1.79356669468566,
0.597231410488591));
#10799=CARTESIAN_POINT('Ctrl Pts',(-0.1269507948667,1.76792916820474,0.587242494443449));
#10800=CARTESIAN_POINT('Ctrl Pts',(-0.154808426054527,1.74874496453875,
0.580140354622989));
#10801=CARTESIAN_POINT('Ctrl Pts',(-0.198771543060865,1.70478184753241,
0.566585944985565));
#10802=CARTESIAN_POINT('Ctrl Pts',(-0.217935681191677,1.67693412158597,
0.559192847558339));
#10803=CARTESIAN_POINT('Ctrl Pts',(-0.243557727551164,1.61548166177648,
0.548518231057014));
#10804=CARTESIAN_POINT('Ctrl Pts',(-0.25,1.58183602855499,0.545435605731786));
#10805=CARTESIAN_POINT('Ctrl Pts',(-0.25,1.55,0.545435605731786));
#10806=CARTESIAN_POINT('',(-0.25,1.55,0.));
#10807=CARTESIAN_POINT('Origin',(1.65,2.25,0.));
#10808=CARTESIAN_POINT('',(-0.6,2.25,-7.34788079488412E-17));
#10809=CARTESIAN_POINT('Origin',(0.,2.25,0.));
#10810=CARTESIAN_POINT('Origin',(1.75,0.85,0.));
#10811=CARTESIAN_POINT('',(-1.75,0.85,-2.14313189850787E-16));
#10812=CARTESIAN_POINT('Origin',(0.,0.85,0.));
#10813=CARTESIAN_POINT('Origin',(0.,0.,0.));
#10814=CARTESIAN_POINT('',(-1.75,-0.85,-2.14313189850787E-16));
#10815=CARTESIAN_POINT('Origin',(0.,-0.85,0.));
#10816=CARTESIAN_POINT('',(-1.75,0.,-2.14313189850787E-16));
#10817=CARTESIAN_POINT('Origin',(0.6,-0.85,0.));
#10818=CARTESIAN_POINT('',(-0.6,-0.85,-7.34788079488412E-17));
#10819=CARTESIAN_POINT('Origin',(0.,-0.85,0.));
#10820=CARTESIAN_POINT('Origin',(0.,0.7,0.));
#10821=CARTESIAN_POINT('',(-0.6,0.7,-7.34788079488412E-17));
#11509=UNCERTAINTY_MEASURE_WITH_UNIT(LENGTH_MEASURE(0.001),#11560,
'DISTANCE_ACCURACY_VALUE',
'Maximum model space distance between geometric entities at asserted c
onnectivities');
#11522=UNCERTAINTY_MEASURE_WITH_UNIT(LENGTH_MEASURE(0.001),#11560,
'DISTANCE_ACCURACY_VALUE',
'Maximum model space distance between geometric entities at asserted c
onnectivities');
#11546=(
GEOMETRIC_REPRESENTATION_CONTEXT(3)
GLOBAL_UNCERTAINTY_ASSIGNED_CONTEXT((#11509))
GLOBAL_UNIT_ASSIGNED_CONTEXT((#11560,#11562,#11563))
REPRESENTATION_CONTEXT('','3D')
);
#11559=(
GEOMETRIC_REPRESENTATION_CONTEXT(3)
GLOBAL_UNCERTAINTY_ASSIGNED_CONTEXT((#11522))
GLOBAL_UNIT_ASSIGNED_CONTEXT((#11560,#11562,#11563))
REPRESENTATION_CONTEXT('','3D')
);
#11560=(
LENGTH_UNIT()
NAMED_UNIT(*)
SI_UNIT(.CENTI.,.METRE.)
);
#11562=(
NAMED_UNIT(*)
PLANE_ANGLE_UNIT()
SI_UNIT($,.RADIAN.)
);
#11563=(
NAMED_UNIT(*)
SI_UNIT($,.STERADIAN.)
SOLID_ANGLE_UNIT()
);
#11587=SHAPE_DEFINITION_REPRESENTATION(#11623,#11744);
#11623=PRODUCT_DEFINITION_SHAPE('',$,#11781);
#11744=SHAPE_REPRESENTATION('',(#7077),#11546);
#11757=PRODUCT_DEFINITION_CONTEXT('part definition',#11867,'design');
#11781=PRODUCT_DEFINITION('Insert bearing','Insert bearing',#11817,#11757);
#11817=PRODUCT_DEFINITION_FORMATION('',$,#11892);
#11867=APPLICATION_CONTEXT(
'Core Data for Automotive Mechanical Design Process');
#11868=PRODUCT_CONTEXT('part definition',#11867,'mechanical');
#11892=PRODUCT('Insert bearing','Insert bearing','Insert bearing',(#11868));
#11961=COLOUR_RGB('Grey',0.48,0.52,0.57);
#11962=FILL_AREA_STYLE_COLOUR('',#11961);
#11963=FILL_AREA_STYLE('',(#11962));
#11964=SURFACE_STYLE_FILL_AREA(#11963);
#11965=SURFACE_SIDE_STYLE('',(#11964));
#11966=SURFACE_STYLE_USAGE(.BOTH.,#11965);
#11967=PRESENTATION_STYLE_ASSIGNMENT((#11966));
ENDSEC;
END-ISO-10303-21;
